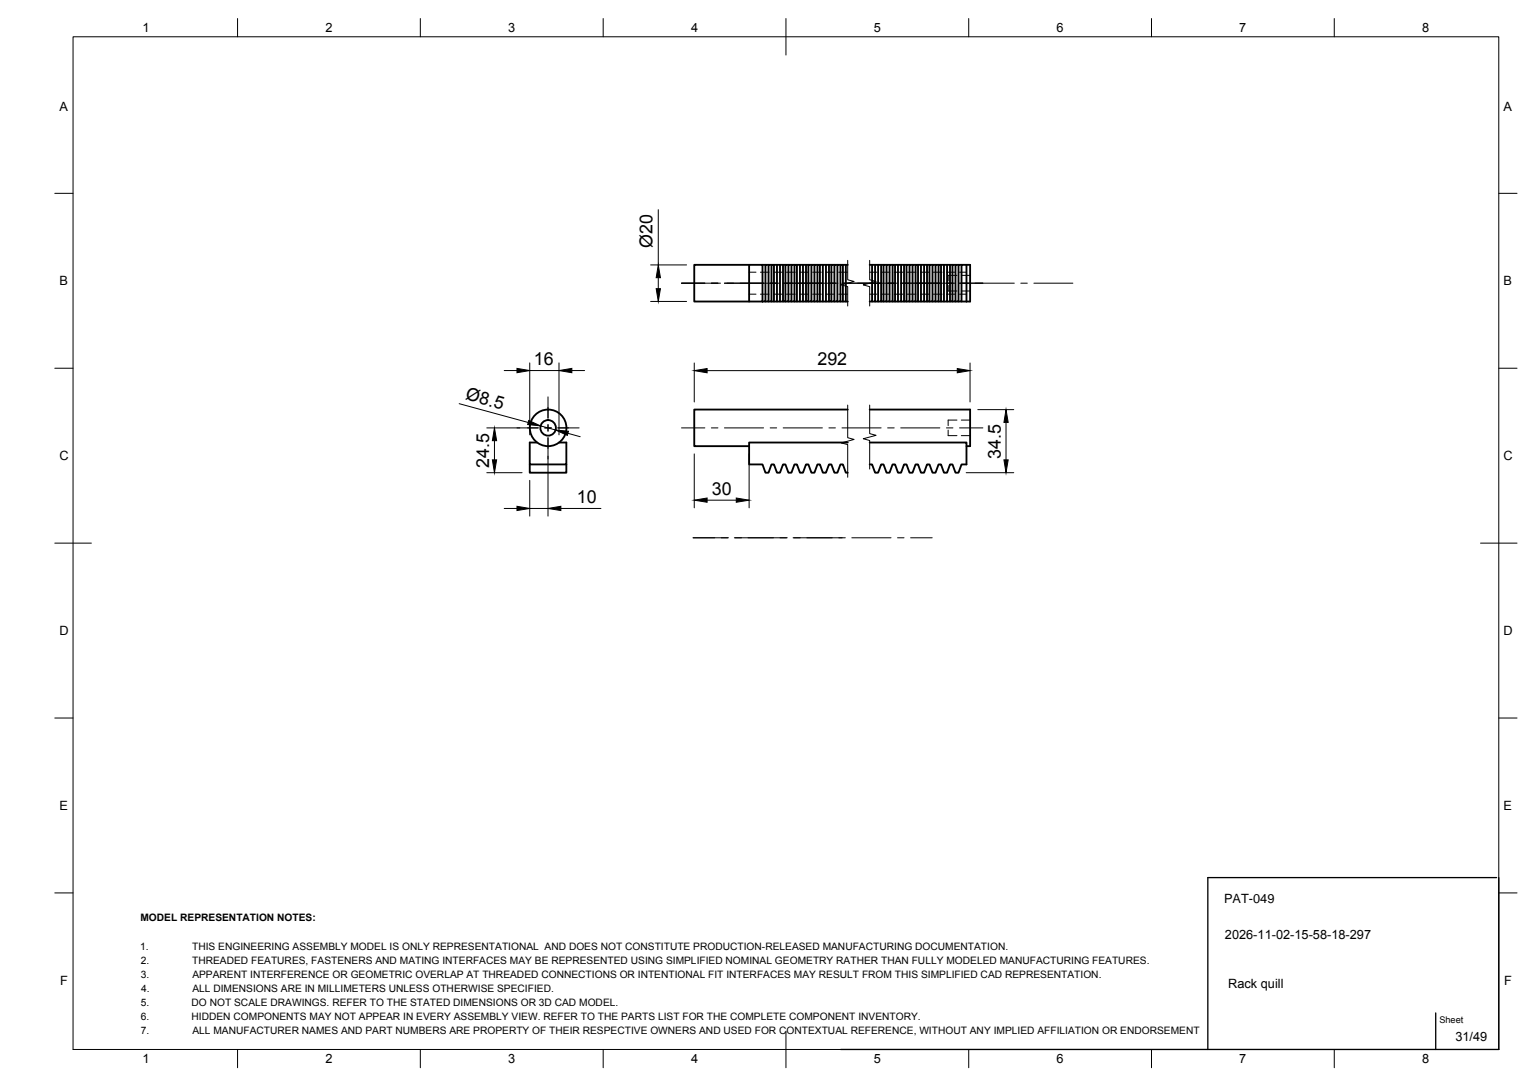
ISO-10303-21;
HEADER;
/* Generated by software containing ST-Developer
 * from STEP Tools, Inc. (www.steptools.com) 
 */

FILE_DESCRIPTION(
/* description */ ('Hand drill press frame (manual)'),
/* implementation_level */ '2;1');

FILE_NAME(
/* name */ 'Rack quill.step',
/* time_stamp */ '2026-10-28T03:25:28-07:00',
/* author */ (''),
/* organization */ (''),
/* preprocessor_version */ 'ST-DEVELOPER v20.2',
/* originating_system */ 'Autodesk Translation Framework v15.17.0.0',
/* authorisation */ '');

FILE_SCHEMA (('AUTOMOTIVE_DESIGN { 1 0 10303 214 3 1 1 }'));
ENDSEC;

DATA;
#10=MECHANICAL_DESIGN_GEOMETRIC_PRESENTATION_REPRESENTATION('',(#649),#33299);
#552=SHAPE_REPRESENTATION_RELATIONSHIP('SRR','None',#33513,#597);
#597=ADVANCED_BREP_SHAPE_REPRESENTATION('',(#700),#33275);
#649=STYLED_ITEM('',(#33800),#700);
#700=MANIFOLD_SOLID_BREP('Body1',#12668);
#846=FACE_BOUND('',#2607,.T.);
#1044=PLANE('',#13760);
#1045=PLANE('',#13761);
#1046=PLANE('',#13762);
#1047=PLANE('',#13763);
#1048=PLANE('',#13766);
#1049=PLANE('',#13769);
#1050=PLANE('',#13770);
#1051=PLANE('',#13771);
#1052=PLANE('',#13772);
#1053=PLANE('',#13773);
#1054=PLANE('',#13774);
#1055=PLANE('',#13775);
#1056=PLANE('',#13776);
#1057=PLANE('',#13777);
#1058=PLANE('',#13778);
#1059=PLANE('',#13779);
#1060=PLANE('',#13780);
#1061=PLANE('',#13781);
#1062=PLANE('',#13782);
#1063=PLANE('',#13783);
#1064=PLANE('',#13784);
#1065=PLANE('',#13785);
#1066=PLANE('',#13786);
#1067=PLANE('',#13787);
#1068=PLANE('',#13788);
#1069=PLANE('',#13789);
#1070=PLANE('',#13790);
#1071=PLANE('',#13791);
#1072=PLANE('',#13792);
#1073=PLANE('',#13793);
#1074=PLANE('',#13794);
#1075=PLANE('',#13795);
#1076=PLANE('',#13796);
#1077=PLANE('',#13797);
#1078=PLANE('',#13798);
#1079=PLANE('',#13799);
#1080=PLANE('',#13800);
#1081=PLANE('',#13801);
#1082=PLANE('',#13802);
#1083=PLANE('',#13803);
#1084=PLANE('',#13804);
#1085=PLANE('',#13805);
#1086=PLANE('',#13806);
#1087=PLANE('',#13807);
#1088=PLANE('',#13808);
#1089=PLANE('',#13809);
#1090=PLANE('',#13810);
#1091=PLANE('',#13811);
#1092=PLANE('',#13812);
#1093=PLANE('',#13813);
#1094=PLANE('',#13814);
#1095=PLANE('',#13815);
#1096=PLANE('',#13816);
#1097=PLANE('',#13817);
#1098=PLANE('',#13818);
#1099=PLANE('',#13819);
#1100=PLANE('',#13820);
#1101=PLANE('',#13821);
#1102=PLANE('',#13822);
#1103=PLANE('',#13823);
#1104=PLANE('',#13824);
#1105=PLANE('',#13825);
#1106=PLANE('',#13826);
#1107=PLANE('',#13827);
#1108=PLANE('',#13828);
#1109=PLANE('',#13829);
#1110=PLANE('',#13830);
#1111=PLANE('',#13831);
#1112=PLANE('',#13832);
#1113=PLANE('',#13833);
#1114=PLANE('',#13834);
#1115=PLANE('',#13835);
#1116=PLANE('',#13836);
#1117=PLANE('',#13837);
#1118=PLANE('',#13838);
#1119=PLANE('',#13839);
#1120=PLANE('',#13840);
#1121=PLANE('',#13841);
#1122=PLANE('',#13842);
#1123=PLANE('',#13843);
#1124=PLANE('',#13844);
#1125=PLANE('',#13845);
#1126=PLANE('',#13846);
#1127=PLANE('',#13847);
#1128=PLANE('',#13848);
#1129=PLANE('',#13849);
#1130=PLANE('',#13850);
#1131=PLANE('',#13851);
#1132=PLANE('',#13852);
#1133=PLANE('',#13853);
#1134=PLANE('',#13854);
#1135=PLANE('',#13855);
#1136=PLANE('',#13856);
#1137=PLANE('',#13857);
#1138=PLANE('',#13858);
#1139=PLANE('',#13859);
#1140=PLANE('',#13860);
#1141=PLANE('',#13861);
#1142=PLANE('',#13862);
#1143=PLANE('',#13863);
#1144=PLANE('',#13864);
#1145=PLANE('',#13865);
#1146=PLANE('',#13866);
#1147=PLANE('',#13867);
#1148=PLANE('',#13868);
#1149=PLANE('',#13869);
#1150=PLANE('',#13870);
#1151=PLANE('',#13871);
#1152=PLANE('',#13872);
#1153=PLANE('',#13873);
#1154=PLANE('',#13874);
#1155=PLANE('',#13875);
#1156=PLANE('',#13876);
#1157=PLANE('',#13877);
#1158=PLANE('',#13878);
#1159=PLANE('',#13879);
#1160=PLANE('',#13880);
#1161=PLANE('',#13881);
#1162=PLANE('',#13882);
#1163=PLANE('',#13883);
#1164=PLANE('',#13884);
#1165=PLANE('',#13885);
#1166=PLANE('',#13886);
#1167=PLANE('',#13887);
#1168=PLANE('',#13888);
#1169=PLANE('',#13889);
#1170=PLANE('',#13890);
#1171=PLANE('',#13891);
#1172=PLANE('',#13892);
#1173=PLANE('',#13893);
#1174=PLANE('',#13894);
#1175=PLANE('',#13895);
#1176=PLANE('',#13896);
#1177=PLANE('',#13897);
#1178=PLANE('',#13898);
#1179=PLANE('',#13899);
#1180=PLANE('',#13900);
#1181=PLANE('',#13901);
#1182=PLANE('',#13902);
#1183=PLANE('',#13903);
#1184=PLANE('',#13904);
#1185=PLANE('',#13905);
#1186=PLANE('',#13906);
#1187=PLANE('',#13907);
#1188=PLANE('',#13908);
#1189=PLANE('',#13909);
#1190=PLANE('',#13910);
#1191=PLANE('',#13911);
#1192=PLANE('',#13912);
#1193=PLANE('',#13913);
#1194=PLANE('',#13914);
#1195=PLANE('',#13915);
#1196=PLANE('',#13916);
#1197=PLANE('',#13917);
#1198=PLANE('',#13918);
#1199=PLANE('',#13919);
#1200=PLANE('',#13920);
#1201=PLANE('',#13921);
#1202=PLANE('',#13922);
#1203=PLANE('',#13923);
#1204=PLANE('',#13924);
#1205=PLANE('',#13925);
#1206=PLANE('',#13926);
#1207=PLANE('',#13927);
#1208=PLANE('',#13928);
#1209=PLANE('',#13929);
#1210=PLANE('',#13930);
#1211=PLANE('',#13931);
#1212=PLANE('',#13935);
#1213=PLANE('',#13936);
#1620=FACE_OUTER_BOUND('',#2435,.T.);
#1621=FACE_OUTER_BOUND('',#2436,.T.);
#1622=FACE_OUTER_BOUND('',#2437,.T.);
#1623=FACE_OUTER_BOUND('',#2438,.T.);
#1624=FACE_OUTER_BOUND('',#2439,.T.);
#1625=FACE_OUTER_BOUND('',#2440,.T.);
#1626=FACE_OUTER_BOUND('',#2441,.T.);
#1627=FACE_OUTER_BOUND('',#2442,.T.);
#1628=FACE_OUTER_BOUND('',#2443,.T.);
#1629=FACE_OUTER_BOUND('',#2444,.T.);
#1630=FACE_OUTER_BOUND('',#2445,.T.);
#1631=FACE_OUTER_BOUND('',#2446,.T.);
#1632=FACE_OUTER_BOUND('',#2447,.T.);
#1633=FACE_OUTER_BOUND('',#2448,.T.);
#1634=FACE_OUTER_BOUND('',#2449,.T.);
#1635=FACE_OUTER_BOUND('',#2450,.T.);
#1636=FACE_OUTER_BOUND('',#2451,.T.);
#1637=FACE_OUTER_BOUND('',#2452,.T.);
#1638=FACE_OUTER_BOUND('',#2453,.T.);
#1639=FACE_OUTER_BOUND('',#2454,.T.);
#1640=FACE_OUTER_BOUND('',#2455,.T.);
#1641=FACE_OUTER_BOUND('',#2456,.T.);
#1642=FACE_OUTER_BOUND('',#2457,.T.);
#1643=FACE_OUTER_BOUND('',#2458,.T.);
#1644=FACE_OUTER_BOUND('',#2459,.T.);
#1645=FACE_OUTER_BOUND('',#2460,.T.);
#1646=FACE_OUTER_BOUND('',#2461,.T.);
#1647=FACE_OUTER_BOUND('',#2462,.T.);
#1648=FACE_OUTER_BOUND('',#2463,.T.);
#1649=FACE_OUTER_BOUND('',#2464,.T.);
#1650=FACE_OUTER_BOUND('',#2465,.T.);
#1651=FACE_OUTER_BOUND('',#2466,.T.);
#1652=FACE_OUTER_BOUND('',#2467,.T.);
#1653=FACE_OUTER_BOUND('',#2468,.T.);
#1654=FACE_OUTER_BOUND('',#2469,.T.);
#1655=FACE_OUTER_BOUND('',#2470,.T.);
#1656=FACE_OUTER_BOUND('',#2471,.T.);
#1657=FACE_OUTER_BOUND('',#2472,.T.);
#1658=FACE_OUTER_BOUND('',#2473,.T.);
#1659=FACE_OUTER_BOUND('',#2474,.T.);
#1660=FACE_OUTER_BOUND('',#2475,.T.);
#1661=FACE_OUTER_BOUND('',#2476,.T.);
#1662=FACE_OUTER_BOUND('',#2477,.T.);
#1663=FACE_OUTER_BOUND('',#2478,.T.);
#1664=FACE_OUTER_BOUND('',#2479,.T.);
#1665=FACE_OUTER_BOUND('',#2480,.T.);
#1666=FACE_OUTER_BOUND('',#2481,.T.);
#1667=FACE_OUTER_BOUND('',#2482,.T.);
#1668=FACE_OUTER_BOUND('',#2483,.T.);
#1669=FACE_OUTER_BOUND('',#2484,.T.);
#1670=FACE_OUTER_BOUND('',#2485,.T.);
#1671=FACE_OUTER_BOUND('',#2486,.T.);
#1672=FACE_OUTER_BOUND('',#2487,.T.);
#1673=FACE_OUTER_BOUND('',#2488,.T.);
#1674=FACE_OUTER_BOUND('',#2489,.T.);
#1675=FACE_OUTER_BOUND('',#2490,.T.);
#1676=FACE_OUTER_BOUND('',#2491,.T.);
#1677=FACE_OUTER_BOUND('',#2492,.T.);
#1678=FACE_OUTER_BOUND('',#2493,.T.);
#1679=FACE_OUTER_BOUND('',#2494,.T.);
#1680=FACE_OUTER_BOUND('',#2495,.T.);
#1681=FACE_OUTER_BOUND('',#2496,.T.);
#1682=FACE_OUTER_BOUND('',#2497,.T.);
#1683=FACE_OUTER_BOUND('',#2498,.T.);
#1684=FACE_OUTER_BOUND('',#2499,.T.);
#1685=FACE_OUTER_BOUND('',#2500,.T.);
#1686=FACE_OUTER_BOUND('',#2501,.T.);
#1687=FACE_OUTER_BOUND('',#2502,.T.);
#1688=FACE_OUTER_BOUND('',#2503,.T.);
#1689=FACE_OUTER_BOUND('',#2504,.T.);
#1690=FACE_OUTER_BOUND('',#2505,.T.);
#1691=FACE_OUTER_BOUND('',#2506,.T.);
#1692=FACE_OUTER_BOUND('',#2507,.T.);
#1693=FACE_OUTER_BOUND('',#2508,.T.);
#1694=FACE_OUTER_BOUND('',#2509,.T.);
#1695=FACE_OUTER_BOUND('',#2510,.T.);
#1696=FACE_OUTER_BOUND('',#2511,.T.);
#1697=FACE_OUTER_BOUND('',#2512,.T.);
#1698=FACE_OUTER_BOUND('',#2513,.T.);
#1699=FACE_OUTER_BOUND('',#2514,.T.);
#1700=FACE_OUTER_BOUND('',#2515,.T.);
#1701=FACE_OUTER_BOUND('',#2516,.T.);
#1702=FACE_OUTER_BOUND('',#2517,.T.);
#1703=FACE_OUTER_BOUND('',#2518,.T.);
#1704=FACE_OUTER_BOUND('',#2519,.T.);
#1705=FACE_OUTER_BOUND('',#2520,.T.);
#1706=FACE_OUTER_BOUND('',#2521,.T.);
#1707=FACE_OUTER_BOUND('',#2522,.T.);
#1708=FACE_OUTER_BOUND('',#2523,.T.);
#1709=FACE_OUTER_BOUND('',#2524,.T.);
#1710=FACE_OUTER_BOUND('',#2525,.T.);
#1711=FACE_OUTER_BOUND('',#2526,.T.);
#1712=FACE_OUTER_BOUND('',#2527,.T.);
#1713=FACE_OUTER_BOUND('',#2528,.T.);
#1714=FACE_OUTER_BOUND('',#2529,.T.);
#1715=FACE_OUTER_BOUND('',#2530,.T.);
#1716=FACE_OUTER_BOUND('',#2531,.T.);
#1717=FACE_OUTER_BOUND('',#2532,.T.);
#1718=FACE_OUTER_BOUND('',#2533,.T.);
#1719=FACE_OUTER_BOUND('',#2534,.T.);
#1720=FACE_OUTER_BOUND('',#2535,.T.);
#1721=FACE_OUTER_BOUND('',#2536,.T.);
#1722=FACE_OUTER_BOUND('',#2537,.T.);
#1723=FACE_OUTER_BOUND('',#2538,.T.);
#1724=FACE_OUTER_BOUND('',#2539,.T.);
#1725=FACE_OUTER_BOUND('',#2540,.T.);
#1726=FACE_OUTER_BOUND('',#2541,.T.);
#1727=FACE_OUTER_BOUND('',#2542,.T.);
#1728=FACE_OUTER_BOUND('',#2543,.T.);
#1729=FACE_OUTER_BOUND('',#2544,.T.);
#1730=FACE_OUTER_BOUND('',#2545,.T.);
#1731=FACE_OUTER_BOUND('',#2546,.T.);
#1732=FACE_OUTER_BOUND('',#2547,.T.);
#1733=FACE_OUTER_BOUND('',#2548,.T.);
#1734=FACE_OUTER_BOUND('',#2549,.T.);
#1735=FACE_OUTER_BOUND('',#2550,.T.);
#1736=FACE_OUTER_BOUND('',#2551,.T.);
#1737=FACE_OUTER_BOUND('',#2552,.T.);
#1738=FACE_OUTER_BOUND('',#2553,.T.);
#1739=FACE_OUTER_BOUND('',#2554,.T.);
#1740=FACE_OUTER_BOUND('',#2555,.T.);
#1741=FACE_OUTER_BOUND('',#2556,.T.);
#1742=FACE_OUTER_BOUND('',#2557,.T.);
#1743=FACE_OUTER_BOUND('',#2558,.T.);
#1744=FACE_OUTER_BOUND('',#2559,.T.);
#1745=FACE_OUTER_BOUND('',#2560,.T.);
#1746=FACE_OUTER_BOUND('',#2561,.T.);
#1747=FACE_OUTER_BOUND('',#2562,.T.);
#1748=FACE_OUTER_BOUND('',#2563,.T.);
#1749=FACE_OUTER_BOUND('',#2564,.T.);
#1750=FACE_OUTER_BOUND('',#2565,.T.);
#1751=FACE_OUTER_BOUND('',#2566,.T.);
#1752=FACE_OUTER_BOUND('',#2567,.T.);
#1753=FACE_OUTER_BOUND('',#2568,.T.);
#1754=FACE_OUTER_BOUND('',#2569,.T.);
#1755=FACE_OUTER_BOUND('',#2570,.T.);
#1756=FACE_OUTER_BOUND('',#2571,.T.);
#1757=FACE_OUTER_BOUND('',#2572,.T.);
#1758=FACE_OUTER_BOUND('',#2573,.T.);
#1759=FACE_OUTER_BOUND('',#2574,.T.);
#1760=FACE_OUTER_BOUND('',#2575,.T.);
#1761=FACE_OUTER_BOUND('',#2576,.T.);
#1762=FACE_OUTER_BOUND('',#2577,.T.);
#1763=FACE_OUTER_BOUND('',#2578,.T.);
#1764=FACE_OUTER_BOUND('',#2579,.T.);
#1765=FACE_OUTER_BOUND('',#2580,.T.);
#1766=FACE_OUTER_BOUND('',#2581,.T.);
#1767=FACE_OUTER_BOUND('',#2582,.T.);
#1768=FACE_OUTER_BOUND('',#2583,.T.);
#1769=FACE_OUTER_BOUND('',#2584,.T.);
#1770=FACE_OUTER_BOUND('',#2585,.T.);
#1771=FACE_OUTER_BOUND('',#2586,.T.);
#1772=FACE_OUTER_BOUND('',#2587,.T.);
#1773=FACE_OUTER_BOUND('',#2588,.T.);
#1774=FACE_OUTER_BOUND('',#2589,.T.);
#1775=FACE_OUTER_BOUND('',#2590,.T.);
#1776=FACE_OUTER_BOUND('',#2591,.T.);
#1777=FACE_OUTER_BOUND('',#2592,.T.);
#1778=FACE_OUTER_BOUND('',#2593,.T.);
#1779=FACE_OUTER_BOUND('',#2594,.T.);
#1780=FACE_OUTER_BOUND('',#2595,.T.);
#1781=FACE_OUTER_BOUND('',#2596,.T.);
#1782=FACE_OUTER_BOUND('',#2597,.T.);
#1783=FACE_OUTER_BOUND('',#2598,.T.);
#1784=FACE_OUTER_BOUND('',#2599,.T.);
#1785=FACE_OUTER_BOUND('',#2600,.T.);
#1786=FACE_OUTER_BOUND('',#2601,.T.);
#1787=FACE_OUTER_BOUND('',#2602,.T.);
#1788=FACE_OUTER_BOUND('',#2603,.T.);
#1789=FACE_OUTER_BOUND('',#2604,.T.);
#1790=FACE_OUTER_BOUND('',#2605,.T.);
#1791=FACE_OUTER_BOUND('',#2606,.T.);
#2435=EDGE_LOOP('',(#9705,#9706,#9707,#9708));
#2436=EDGE_LOOP('',(#9709));
#2437=EDGE_LOOP('',(#9710,#9711,#9712,#9713));
#2438=EDGE_LOOP('',(#9714,#9715,#9716,#9717));
#2439=EDGE_LOOP('',(#9718,#9719,#9720,#9721,#9722,#9723,#9724));
#2440=EDGE_LOOP('',(#9725,#9726,#9727,#9728,#9729,#9730,#9731));
#2441=EDGE_LOOP('',(#9732,#9733,#9734,#9735));
#2442=EDGE_LOOP('',(#9736,#9737,#9738,#9739));
#2443=EDGE_LOOP('',(#9740,#9741,#9742,#9743));
#2444=EDGE_LOOP('',(#9744,#9745,#9746,#9747));
#2445=EDGE_LOOP('',(#9748,#9749,#9750,#9751));
#2446=EDGE_LOOP('',(#9752,#9753,#9754,#9755));
#2447=EDGE_LOOP('',(#9756,#9757,#9758,#9759));
#2448=EDGE_LOOP('',(#9760,#9761,#9762,#9763));
#2449=EDGE_LOOP('',(#9764,#9765,#9766,#9767));
#2450=EDGE_LOOP('',(#9768,#9769,#9770,#9771));
#2451=EDGE_LOOP('',(#9772,#9773,#9774,#9775));
#2452=EDGE_LOOP('',(#9776,#9777,#9778,#9779));
#2453=EDGE_LOOP('',(#9780,#9781,#9782,#9783));
#2454=EDGE_LOOP('',(#9784,#9785,#9786,#9787));
#2455=EDGE_LOOP('',(#9788,#9789,#9790,#9791));
#2456=EDGE_LOOP('',(#9792,#9793,#9794,#9795));
#2457=EDGE_LOOP('',(#9796,#9797,#9798,#9799));
#2458=EDGE_LOOP('',(#9800,#9801,#9802,#9803));
#2459=EDGE_LOOP('',(#9804,#9805,#9806,#9807));
#2460=EDGE_LOOP('',(#9808,#9809,#9810,#9811));
#2461=EDGE_LOOP('',(#9812,#9813,#9814,#9815));
#2462=EDGE_LOOP('',(#9816,#9817,#9818,#9819));
#2463=EDGE_LOOP('',(#9820,#9821,#9822,#9823));
#2464=EDGE_LOOP('',(#9824,#9825,#9826,#9827));
#2465=EDGE_LOOP('',(#9828,#9829,#9830,#9831));
#2466=EDGE_LOOP('',(#9832,#9833,#9834,#9835));
#2467=EDGE_LOOP('',(#9836,#9837,#9838,#9839));
#2468=EDGE_LOOP('',(#9840,#9841,#9842,#9843));
#2469=EDGE_LOOP('',(#9844,#9845,#9846,#9847));
#2470=EDGE_LOOP('',(#9848,#9849,#9850,#9851));
#2471=EDGE_LOOP('',(#9852,#9853,#9854,#9855));
#2472=EDGE_LOOP('',(#9856,#9857,#9858,#9859));
#2473=EDGE_LOOP('',(#9860,#9861,#9862,#9863));
#2474=EDGE_LOOP('',(#9864,#9865,#9866,#9867));
#2475=EDGE_LOOP('',(#9868,#9869,#9870,#9871));
#2476=EDGE_LOOP('',(#9872,#9873,#9874,#9875));
#2477=EDGE_LOOP('',(#9876,#9877,#9878,#9879));
#2478=EDGE_LOOP('',(#9880,#9881,#9882,#9883));
#2479=EDGE_LOOP('',(#9884,#9885,#9886,#9887));
#2480=EDGE_LOOP('',(#9888,#9889,#9890,#9891));
#2481=EDGE_LOOP('',(#9892,#9893,#9894,#9895));
#2482=EDGE_LOOP('',(#9896,#9897,#9898,#9899));
#2483=EDGE_LOOP('',(#9900,#9901,#9902,#9903));
#2484=EDGE_LOOP('',(#9904,#9905,#9906,#9907));
#2485=EDGE_LOOP('',(#9908,#9909,#9910,#9911));
#2486=EDGE_LOOP('',(#9912,#9913,#9914,#9915));
#2487=EDGE_LOOP('',(#9916,#9917,#9918,#9919));
#2488=EDGE_LOOP('',(#9920,#9921,#9922,#9923));
#2489=EDGE_LOOP('',(#9924,#9925,#9926,#9927));
#2490=EDGE_LOOP('',(#9928,#9929,#9930,#9931));
#2491=EDGE_LOOP('',(#9932,#9933,#9934,#9935));
#2492=EDGE_LOOP('',(#9936,#9937,#9938,#9939));
#2493=EDGE_LOOP('',(#9940,#9941,#9942,#9943));
#2494=EDGE_LOOP('',(#9944,#9945,#9946,#9947));
#2495=EDGE_LOOP('',(#9948,#9949,#9950,#9951));
#2496=EDGE_LOOP('',(#9952,#9953,#9954,#9955));
#2497=EDGE_LOOP('',(#9956,#9957,#9958,#9959));
#2498=EDGE_LOOP('',(#9960,#9961,#9962,#9963));
#2499=EDGE_LOOP('',(#9964,#9965,#9966,#9967));
#2500=EDGE_LOOP('',(#9968,#9969,#9970,#9971));
#2501=EDGE_LOOP('',(#9972,#9973,#9974,#9975));
#2502=EDGE_LOOP('',(#9976,#9977,#9978,#9979));
#2503=EDGE_LOOP('',(#9980,#9981,#9982,#9983));
#2504=EDGE_LOOP('',(#9984,#9985,#9986,#9987));
#2505=EDGE_LOOP('',(#9988,#9989,#9990,#9991));
#2506=EDGE_LOOP('',(#9992,#9993,#9994,#9995));
#2507=EDGE_LOOP('',(#9996,#9997,#9998,#9999));
#2508=EDGE_LOOP('',(#10000,#10001,#10002,#10003));
#2509=EDGE_LOOP('',(#10004,#10005,#10006,#10007));
#2510=EDGE_LOOP('',(#10008,#10009,#10010,#10011));
#2511=EDGE_LOOP('',(#10012,#10013,#10014,#10015));
#2512=EDGE_LOOP('',(#10016,#10017,#10018,#10019));
#2513=EDGE_LOOP('',(#10020,#10021,#10022,#10023));
#2514=EDGE_LOOP('',(#10024,#10025,#10026,#10027));
#2515=EDGE_LOOP('',(#10028,#10029,#10030,#10031));
#2516=EDGE_LOOP('',(#10032,#10033,#10034,#10035));
#2517=EDGE_LOOP('',(#10036,#10037,#10038,#10039));
#2518=EDGE_LOOP('',(#10040,#10041,#10042,#10043));
#2519=EDGE_LOOP('',(#10044,#10045,#10046,#10047));
#2520=EDGE_LOOP('',(#10048,#10049,#10050,#10051));
#2521=EDGE_LOOP('',(#10052,#10053,#10054,#10055));
#2522=EDGE_LOOP('',(#10056,#10057,#10058,#10059));
#2523=EDGE_LOOP('',(#10060,#10061,#10062,#10063));
#2524=EDGE_LOOP('',(#10064,#10065,#10066,#10067));
#2525=EDGE_LOOP('',(#10068,#10069,#10070,#10071));
#2526=EDGE_LOOP('',(#10072,#10073,#10074,#10075));
#2527=EDGE_LOOP('',(#10076,#10077,#10078,#10079));
#2528=EDGE_LOOP('',(#10080,#10081,#10082,#10083));
#2529=EDGE_LOOP('',(#10084,#10085,#10086,#10087));
#2530=EDGE_LOOP('',(#10088,#10089,#10090,#10091));
#2531=EDGE_LOOP('',(#10092,#10093,#10094,#10095));
#2532=EDGE_LOOP('',(#10096,#10097,#10098,#10099));
#2533=EDGE_LOOP('',(#10100,#10101,#10102,#10103));
#2534=EDGE_LOOP('',(#10104,#10105,#10106,#10107));
#2535=EDGE_LOOP('',(#10108,#10109,#10110,#10111));
#2536=EDGE_LOOP('',(#10112,#10113,#10114,#10115));
#2537=EDGE_LOOP('',(#10116,#10117,#10118,#10119));
#2538=EDGE_LOOP('',(#10120,#10121,#10122,#10123));
#2539=EDGE_LOOP('',(#10124,#10125,#10126,#10127));
#2540=EDGE_LOOP('',(#10128,#10129,#10130,#10131));
#2541=EDGE_LOOP('',(#10132,#10133,#10134,#10135));
#2542=EDGE_LOOP('',(#10136,#10137,#10138,#10139));
#2543=EDGE_LOOP('',(#10140,#10141,#10142,#10143));
#2544=EDGE_LOOP('',(#10144,#10145,#10146,#10147));
#2545=EDGE_LOOP('',(#10148,#10149,#10150,#10151));
#2546=EDGE_LOOP('',(#10152,#10153,#10154,#10155));
#2547=EDGE_LOOP('',(#10156,#10157,#10158,#10159));
#2548=EDGE_LOOP('',(#10160,#10161,#10162,#10163));
#2549=EDGE_LOOP('',(#10164,#10165,#10166,#10167));
#2550=EDGE_LOOP('',(#10168,#10169,#10170,#10171));
#2551=EDGE_LOOP('',(#10172,#10173,#10174,#10175));
#2552=EDGE_LOOP('',(#10176,#10177,#10178,#10179));
#2553=EDGE_LOOP('',(#10180,#10181,#10182,#10183));
#2554=EDGE_LOOP('',(#10184,#10185,#10186,#10187));
#2555=EDGE_LOOP('',(#10188,#10189,#10190,#10191));
#2556=EDGE_LOOP('',(#10192,#10193,#10194,#10195));
#2557=EDGE_LOOP('',(#10196,#10197,#10198,#10199));
#2558=EDGE_LOOP('',(#10200,#10201,#10202,#10203));
#2559=EDGE_LOOP('',(#10204,#10205,#10206,#10207));
#2560=EDGE_LOOP('',(#10208,#10209,#10210,#10211));
#2561=EDGE_LOOP('',(#10212,#10213,#10214,#10215));
#2562=EDGE_LOOP('',(#10216,#10217,#10218,#10219));
#2563=EDGE_LOOP('',(#10220,#10221,#10222,#10223));
#2564=EDGE_LOOP('',(#10224,#10225,#10226,#10227));
#2565=EDGE_LOOP('',(#10228,#10229,#10230,#10231));
#2566=EDGE_LOOP('',(#10232,#10233,#10234,#10235));
#2567=EDGE_LOOP('',(#10236,#10237,#10238,#10239));
#2568=EDGE_LOOP('',(#10240,#10241,#10242,#10243));
#2569=EDGE_LOOP('',(#10244,#10245,#10246,#10247));
#2570=EDGE_LOOP('',(#10248,#10249,#10250,#10251));
#2571=EDGE_LOOP('',(#10252,#10253,#10254,#10255));
#2572=EDGE_LOOP('',(#10256,#10257,#10258,#10259));
#2573=EDGE_LOOP('',(#10260,#10261,#10262,#10263));
#2574=EDGE_LOOP('',(#10264,#10265,#10266,#10267));
#2575=EDGE_LOOP('',(#10268,#10269,#10270,#10271));
#2576=EDGE_LOOP('',(#10272,#10273,#10274,#10275));
#2577=EDGE_LOOP('',(#10276,#10277,#10278,#10279));
#2578=EDGE_LOOP('',(#10280,#10281,#10282,#10283));
#2579=EDGE_LOOP('',(#10284,#10285,#10286,#10287));
#2580=EDGE_LOOP('',(#10288,#10289,#10290,#10291));
#2581=EDGE_LOOP('',(#10292,#10293,#10294,#10295));
#2582=EDGE_LOOP('',(#10296,#10297,#10298,#10299));
#2583=EDGE_LOOP('',(#10300,#10301,#10302,#10303));
#2584=EDGE_LOOP('',(#10304,#10305,#10306,#10307));
#2585=EDGE_LOOP('',(#10308,#10309,#10310,#10311));
#2586=EDGE_LOOP('',(#10312,#10313,#10314,#10315));
#2587=EDGE_LOOP('',(#10316,#10317,#10318,#10319));
#2588=EDGE_LOOP('',(#10320,#10321,#10322,#10323));
#2589=EDGE_LOOP('',(#10324,#10325,#10326,#10327));
#2590=EDGE_LOOP('',(#10328,#10329,#10330,#10331));
#2591=EDGE_LOOP('',(#10332,#10333,#10334,#10335));
#2592=EDGE_LOOP('',(#10336,#10337,#10338,#10339));
#2593=EDGE_LOOP('',(#10340,#10341,#10342,#10343));
#2594=EDGE_LOOP('',(#10344,#10345,#10346,#10347));
#2595=EDGE_LOOP('',(#10348,#10349,#10350,#10351));
#2596=EDGE_LOOP('',(#10352,#10353,#10354,#10355));
#2597=EDGE_LOOP('',(#10356,#10357,#10358,#10359));
#2598=EDGE_LOOP('',(#10360,#10361,#10362,#10363));
#2599=EDGE_LOOP('',(#10364,#10365,#10366,#10367));
#2600=EDGE_LOOP('',(#10368,#10369,#10370,#10371));
#2601=EDGE_LOOP('',(#10372,#10373,#10374,#10375));
#2602=EDGE_LOOP('',(#10376,#10377,#10378,#10379,#10380,#10381,#10382,#10383,
#10384,#10385,#10386,#10387,#10388,#10389,#10390,#10391,#10392,#10393,#10394,
#10395,#10396,#10397,#10398,#10399,#10400,#10401,#10402,#10403,#10404,#10405,
#10406,#10407,#10408,#10409,#10410,#10411,#10412,#10413,#10414,#10415,#10416,
#10417,#10418,#10419,#10420,#10421,#10422,#10423,#10424,#10425,#10426,#10427,
#10428,#10429,#10430,#10431,#10432,#10433,#10434,#10435,#10436,#10437,#10438,
#10439,#10440,#10441,#10442,#10443,#10444,#10445,#10446,#10447,#10448,#10449,
#10450,#10451,#10452,#10453,#10454,#10455,#10456,#10457,#10458,#10459,#10460,
#10461,#10462,#10463,#10464,#10465,#10466,#10467,#10468,#10469,#10470,#10471,
#10472,#10473,#10474,#10475,#10476,#10477,#10478,#10479,#10480,#10481,#10482,
#10483,#10484,#10485,#10486,#10487,#10488,#10489,#10490,#10491,#10492,#10493,
#10494,#10495,#10496,#10497,#10498,#10499,#10500,#10501,#10502,#10503,#10504,
#10505,#10506,#10507,#10508,#10509,#10510,#10511,#10512,#10513,#10514,#10515,
#10516,#10517,#10518,#10519,#10520,#10521,#10522,#10523,#10524,#10525,#10526,
#10527,#10528,#10529,#10530,#10531,#10532,#10533,#10534,#10535,#10536,#10537,
#10538,#10539));
#2603=EDGE_LOOP('',(#10540,#10541,#10542,#10543,#10544,#10545,#10546,#10547,
#10548,#10549,#10550,#10551,#10552,#10553,#10554,#10555,#10556,#10557,#10558,
#10559,#10560,#10561,#10562,#10563,#10564,#10565,#10566,#10567,#10568,#10569,
#10570,#10571,#10572,#10573,#10574,#10575,#10576,#10577,#10578,#10579,#10580,
#10581,#10582,#10583,#10584,#10585,#10586,#10587,#10588,#10589,#10590,#10591,
#10592,#10593,#10594,#10595,#10596,#10597,#10598,#10599,#10600,#10601,#10602,
#10603,#10604,#10605,#10606,#10607,#10608,#10609,#10610,#10611,#10612,#10613,
#10614,#10615,#10616,#10617,#10618,#10619,#10620,#10621,#10622,#10623,#10624,
#10625,#10626,#10627,#10628,#10629,#10630,#10631,#10632,#10633,#10634,#10635,
#10636,#10637,#10638,#10639,#10640,#10641,#10642,#10643,#10644,#10645,#10646,
#10647,#10648,#10649,#10650,#10651,#10652,#10653,#10654,#10655,#10656,#10657,
#10658,#10659,#10660,#10661,#10662,#10663,#10664,#10665,#10666,#10667,#10668,
#10669,#10670,#10671,#10672,#10673,#10674,#10675,#10676,#10677,#10678,#10679,
#10680,#10681,#10682,#10683,#10684,#10685,#10686,#10687,#10688,#10689,#10690,
#10691,#10692,#10693,#10694,#10695,#10696,#10697,#10698,#10699,#10700,#10701,
#10702,#10703));
#2604=EDGE_LOOP('',(#10704,#10705,#10706,#10707,#10708,#10709,#10710,#10711,
#10712,#10713,#10714,#10715));
#2605=EDGE_LOOP('',(#10716));
#2606=EDGE_LOOP('',(#10717));
#2607=EDGE_LOOP('',(#10718));
#3242=LINE('',#19762,#4407);
#3243=LINE('',#19768,#4408);
#3244=LINE('',#19770,#4409);
#3245=LINE('',#19772,#4410);
#3246=LINE('',#19773,#4411);
#3247=LINE('',#19777,#4412);
#3248=LINE('',#19779,#4413);
#3249=LINE('',#19781,#4414);
#3250=LINE('',#19782,#4415);
#3251=LINE('',#19787,#4416);
#3252=LINE('',#19789,#4417);
#3253=LINE('',#19790,#4418);
#3254=LINE('',#19796,#4419);
#3255=LINE('',#19798,#4420);
#3256=LINE('',#19799,#4421);
#3257=LINE('',#19803,#4422);
#3258=LINE('',#19805,#4423);
#3259=LINE('',#19806,#4424);
#3260=LINE('',#19809,#4425);
#3261=LINE('',#19811,#4426);
#3262=LINE('',#19812,#4427);
#3263=LINE('',#19815,#4428);
#3264=LINE('',#19817,#4429);
#3265=LINE('',#19818,#4430);
#3266=LINE('',#19821,#4431);
#3267=LINE('',#19823,#4432);
#3268=LINE('',#19824,#4433);
#3269=LINE('',#19827,#4434);
#3270=LINE('',#19829,#4435);
#3271=LINE('',#19830,#4436);
#3272=LINE('',#19833,#4437);
#3273=LINE('',#19835,#4438);
#3274=LINE('',#19836,#4439);
#3275=LINE('',#19839,#4440);
#3276=LINE('',#19841,#4441);
#3277=LINE('',#19842,#4442);
#3278=LINE('',#19845,#4443);
#3279=LINE('',#19847,#4444);
#3280=LINE('',#19848,#4445);
#3281=LINE('',#19851,#4446);
#3282=LINE('',#19853,#4447);
#3283=LINE('',#19854,#4448);
#3284=LINE('',#19857,#4449);
#3285=LINE('',#19859,#4450);
#3286=LINE('',#19860,#4451);
#3287=LINE('',#19863,#4452);
#3288=LINE('',#19865,#4453);
#3289=LINE('',#19866,#4454);
#3290=LINE('',#19869,#4455);
#3291=LINE('',#19871,#4456);
#3292=LINE('',#19872,#4457);
#3293=LINE('',#19875,#4458);
#3294=LINE('',#19877,#4459);
#3295=LINE('',#19878,#4460);
#3296=LINE('',#19881,#4461);
#3297=LINE('',#19883,#4462);
#3298=LINE('',#19884,#4463);
#3299=LINE('',#19887,#4464);
#3300=LINE('',#19889,#4465);
#3301=LINE('',#19890,#4466);
#3302=LINE('',#19893,#4467);
#3303=LINE('',#19895,#4468);
#3304=LINE('',#19896,#4469);
#3305=LINE('',#19899,#4470);
#3306=LINE('',#19901,#4471);
#3307=LINE('',#19902,#4472);
#3308=LINE('',#19905,#4473);
#3309=LINE('',#19907,#4474);
#3310=LINE('',#19908,#4475);
#3311=LINE('',#19911,#4476);
#3312=LINE('',#19913,#4477);
#3313=LINE('',#19914,#4478);
#3314=LINE('',#19917,#4479);
#3315=LINE('',#19919,#4480);
#3316=LINE('',#19920,#4481);
#3317=LINE('',#19923,#4482);
#3318=LINE('',#19925,#4483);
#3319=LINE('',#19926,#4484);
#3320=LINE('',#19929,#4485);
#3321=LINE('',#19931,#4486);
#3322=LINE('',#19932,#4487);
#3323=LINE('',#19935,#4488);
#3324=LINE('',#19937,#4489);
#3325=LINE('',#19938,#4490);
#3326=LINE('',#19941,#4491);
#3327=LINE('',#19943,#4492);
#3328=LINE('',#19944,#4493);
#3329=LINE('',#19947,#4494);
#3330=LINE('',#19949,#4495);
#3331=LINE('',#19950,#4496);
#3332=LINE('',#19953,#4497);
#3333=LINE('',#19955,#4498);
#3334=LINE('',#19956,#4499);
#3335=LINE('',#19959,#4500);
#3336=LINE('',#19961,#4501);
#3337=LINE('',#19962,#4502);
#3338=LINE('',#19965,#4503);
#3339=LINE('',#19967,#4504);
#3340=LINE('',#19968,#4505);
#3341=LINE('',#19971,#4506);
#3342=LINE('',#19973,#4507);
#3343=LINE('',#19974,#4508);
#3344=LINE('',#19977,#4509);
#3345=LINE('',#19979,#4510);
#3346=LINE('',#19980,#4511);
#3347=LINE('',#19983,#4512);
#3348=LINE('',#19985,#4513);
#3349=LINE('',#19986,#4514);
#3350=LINE('',#19989,#4515);
#3351=LINE('',#19991,#4516);
#3352=LINE('',#19992,#4517);
#3353=LINE('',#19995,#4518);
#3354=LINE('',#19997,#4519);
#3355=LINE('',#19998,#4520);
#3356=LINE('',#20001,#4521);
#3357=LINE('',#20003,#4522);
#3358=LINE('',#20004,#4523);
#3359=LINE('',#20007,#4524);
#3360=LINE('',#20009,#4525);
#3361=LINE('',#20010,#4526);
#3362=LINE('',#20013,#4527);
#3363=LINE('',#20015,#4528);
#3364=LINE('',#20016,#4529);
#3365=LINE('',#20019,#4530);
#3366=LINE('',#20021,#4531);
#3367=LINE('',#20022,#4532);
#3368=LINE('',#20025,#4533);
#3369=LINE('',#20027,#4534);
#3370=LINE('',#20028,#4535);
#3371=LINE('',#20031,#4536);
#3372=LINE('',#20033,#4537);
#3373=LINE('',#20034,#4538);
#3374=LINE('',#20037,#4539);
#3375=LINE('',#20039,#4540);
#3376=LINE('',#20040,#4541);
#3377=LINE('',#20043,#4542);
#3378=LINE('',#20045,#4543);
#3379=LINE('',#20046,#4544);
#3380=LINE('',#20049,#4545);
#3381=LINE('',#20051,#4546);
#3382=LINE('',#20052,#4547);
#3383=LINE('',#20055,#4548);
#3384=LINE('',#20057,#4549);
#3385=LINE('',#20058,#4550);
#3386=LINE('',#20061,#4551);
#3387=LINE('',#20063,#4552);
#3388=LINE('',#20064,#4553);
#3389=LINE('',#20067,#4554);
#3390=LINE('',#20069,#4555);
#3391=LINE('',#20070,#4556);
#3392=LINE('',#20073,#4557);
#3393=LINE('',#20075,#4558);
#3394=LINE('',#20076,#4559);
#3395=LINE('',#20079,#4560);
#3396=LINE('',#20081,#4561);
#3397=LINE('',#20082,#4562);
#3398=LINE('',#20085,#4563);
#3399=LINE('',#20087,#4564);
#3400=LINE('',#20088,#4565);
#3401=LINE('',#20091,#4566);
#3402=LINE('',#20093,#4567);
#3403=LINE('',#20094,#4568);
#3404=LINE('',#20097,#4569);
#3405=LINE('',#20099,#4570);
#3406=LINE('',#20100,#4571);
#3407=LINE('',#20103,#4572);
#3408=LINE('',#20105,#4573);
#3409=LINE('',#20106,#4574);
#3410=LINE('',#20109,#4575);
#3411=LINE('',#20111,#4576);
#3412=LINE('',#20112,#4577);
#3413=LINE('',#20115,#4578);
#3414=LINE('',#20117,#4579);
#3415=LINE('',#20118,#4580);
#3416=LINE('',#20121,#4581);
#3417=LINE('',#20123,#4582);
#3418=LINE('',#20124,#4583);
#3419=LINE('',#20127,#4584);
#3420=LINE('',#20129,#4585);
#3421=LINE('',#20130,#4586);
#3422=LINE('',#20133,#4587);
#3423=LINE('',#20135,#4588);
#3424=LINE('',#20136,#4589);
#3425=LINE('',#20139,#4590);
#3426=LINE('',#20141,#4591);
#3427=LINE('',#20142,#4592);
#3428=LINE('',#20145,#4593);
#3429=LINE('',#20147,#4594);
#3430=LINE('',#20148,#4595);
#3431=LINE('',#20151,#4596);
#3432=LINE('',#20153,#4597);
#3433=LINE('',#20154,#4598);
#3434=LINE('',#20157,#4599);
#3435=LINE('',#20159,#4600);
#3436=LINE('',#20160,#4601);
#3437=LINE('',#20163,#4602);
#3438=LINE('',#20165,#4603);
#3439=LINE('',#20166,#4604);
#3440=LINE('',#20169,#4605);
#3441=LINE('',#20171,#4606);
#3442=LINE('',#20172,#4607);
#3443=LINE('',#20175,#4608);
#3444=LINE('',#20177,#4609);
#3445=LINE('',#20178,#4610);
#3446=LINE('',#20181,#4611);
#3447=LINE('',#20183,#4612);
#3448=LINE('',#20184,#4613);
#3449=LINE('',#20187,#4614);
#3450=LINE('',#20189,#4615);
#3451=LINE('',#20190,#4616);
#3452=LINE('',#20193,#4617);
#3453=LINE('',#20195,#4618);
#3454=LINE('',#20196,#4619);
#3455=LINE('',#20199,#4620);
#3456=LINE('',#20201,#4621);
#3457=LINE('',#20202,#4622);
#3458=LINE('',#20205,#4623);
#3459=LINE('',#20207,#4624);
#3460=LINE('',#20208,#4625);
#3461=LINE('',#20211,#4626);
#3462=LINE('',#20213,#4627);
#3463=LINE('',#20214,#4628);
#3464=LINE('',#20217,#4629);
#3465=LINE('',#20219,#4630);
#3466=LINE('',#20220,#4631);
#3467=LINE('',#20223,#4632);
#3468=LINE('',#20225,#4633);
#3469=LINE('',#20226,#4634);
#3470=LINE('',#20229,#4635);
#3471=LINE('',#20231,#4636);
#3472=LINE('',#20232,#4637);
#3473=LINE('',#20235,#4638);
#3474=LINE('',#20237,#4639);
#3475=LINE('',#20238,#4640);
#3476=LINE('',#20241,#4641);
#3477=LINE('',#20243,#4642);
#3478=LINE('',#20244,#4643);
#3479=LINE('',#20247,#4644);
#3480=LINE('',#20249,#4645);
#3481=LINE('',#20250,#4646);
#3482=LINE('',#20253,#4647);
#3483=LINE('',#20255,#4648);
#3484=LINE('',#20256,#4649);
#3485=LINE('',#20259,#4650);
#3486=LINE('',#20261,#4651);
#3487=LINE('',#20262,#4652);
#3488=LINE('',#20265,#4653);
#3489=LINE('',#20267,#4654);
#3490=LINE('',#20268,#4655);
#3491=LINE('',#20271,#4656);
#3492=LINE('',#20273,#4657);
#3493=LINE('',#20274,#4658);
#3494=LINE('',#20277,#4659);
#3495=LINE('',#20279,#4660);
#3496=LINE('',#20280,#4661);
#3497=LINE('',#20283,#4662);
#3498=LINE('',#20285,#4663);
#3499=LINE('',#20286,#4664);
#3500=LINE('',#20289,#4665);
#3501=LINE('',#20291,#4666);
#3502=LINE('',#20292,#4667);
#3503=LINE('',#20295,#4668);
#3504=LINE('',#20297,#4669);
#3505=LINE('',#20298,#4670);
#3506=LINE('',#20301,#4671);
#3507=LINE('',#20303,#4672);
#3508=LINE('',#20304,#4673);
#3509=LINE('',#20307,#4674);
#3510=LINE('',#20309,#4675);
#3511=LINE('',#20310,#4676);
#3512=LINE('',#20313,#4677);
#3513=LINE('',#20315,#4678);
#3514=LINE('',#20316,#4679);
#3515=LINE('',#20319,#4680);
#3516=LINE('',#20321,#4681);
#3517=LINE('',#20322,#4682);
#3518=LINE('',#20325,#4683);
#3519=LINE('',#20327,#4684);
#3520=LINE('',#20328,#4685);
#3521=LINE('',#20331,#4686);
#3522=LINE('',#20333,#4687);
#3523=LINE('',#20334,#4688);
#3524=LINE('',#20337,#4689);
#3525=LINE('',#20339,#4690);
#3526=LINE('',#20340,#4691);
#3527=LINE('',#20343,#4692);
#3528=LINE('',#20345,#4693);
#3529=LINE('',#20346,#4694);
#3530=LINE('',#20349,#4695);
#3531=LINE('',#20351,#4696);
#3532=LINE('',#20352,#4697);
#3533=LINE('',#20355,#4698);
#3534=LINE('',#20357,#4699);
#3535=LINE('',#20358,#4700);
#3536=LINE('',#20361,#4701);
#3537=LINE('',#20363,#4702);
#3538=LINE('',#20364,#4703);
#3539=LINE('',#20367,#4704);
#3540=LINE('',#20369,#4705);
#3541=LINE('',#20370,#4706);
#3542=LINE('',#20373,#4707);
#3543=LINE('',#20375,#4708);
#3544=LINE('',#20376,#4709);
#3545=LINE('',#20379,#4710);
#3546=LINE('',#20381,#4711);
#3547=LINE('',#20382,#4712);
#3548=LINE('',#20385,#4713);
#3549=LINE('',#20387,#4714);
#3550=LINE('',#20388,#4715);
#3551=LINE('',#20391,#4716);
#3552=LINE('',#20393,#4717);
#3553=LINE('',#20394,#4718);
#3554=LINE('',#20397,#4719);
#3555=LINE('',#20399,#4720);
#3556=LINE('',#20400,#4721);
#3557=LINE('',#20403,#4722);
#3558=LINE('',#20405,#4723);
#3559=LINE('',#20406,#4724);
#3560=LINE('',#20409,#4725);
#3561=LINE('',#20411,#4726);
#3562=LINE('',#20412,#4727);
#3563=LINE('',#20415,#4728);
#3564=LINE('',#20417,#4729);
#3565=LINE('',#20418,#4730);
#3566=LINE('',#20421,#4731);
#3567=LINE('',#20423,#4732);
#3568=LINE('',#20424,#4733);
#3569=LINE('',#20427,#4734);
#3570=LINE('',#20429,#4735);
#3571=LINE('',#20430,#4736);
#3572=LINE('',#20433,#4737);
#3573=LINE('',#20435,#4738);
#3574=LINE('',#20436,#4739);
#3575=LINE('',#20439,#4740);
#3576=LINE('',#20441,#4741);
#3577=LINE('',#20442,#4742);
#3578=LINE('',#20445,#4743);
#3579=LINE('',#20447,#4744);
#3580=LINE('',#20448,#4745);
#3581=LINE('',#20451,#4746);
#3582=LINE('',#20453,#4747);
#3583=LINE('',#20454,#4748);
#3584=LINE('',#20457,#4749);
#3585=LINE('',#20459,#4750);
#3586=LINE('',#20460,#4751);
#3587=LINE('',#20463,#4752);
#3588=LINE('',#20465,#4753);
#3589=LINE('',#20466,#4754);
#3590=LINE('',#20469,#4755);
#3591=LINE('',#20471,#4756);
#3592=LINE('',#20472,#4757);
#3593=LINE('',#20475,#4758);
#3594=LINE('',#20477,#4759);
#3595=LINE('',#20478,#4760);
#3596=LINE('',#20481,#4761);
#3597=LINE('',#20483,#4762);
#3598=LINE('',#20484,#4763);
#3599=LINE('',#20487,#4764);
#3600=LINE('',#20489,#4765);
#3601=LINE('',#20490,#4766);
#3602=LINE('',#20493,#4767);
#3603=LINE('',#20495,#4768);
#3604=LINE('',#20496,#4769);
#3605=LINE('',#20499,#4770);
#3606=LINE('',#20501,#4771);
#3607=LINE('',#20502,#4772);
#3608=LINE('',#20505,#4773);
#3609=LINE('',#20507,#4774);
#3610=LINE('',#20508,#4775);
#3611=LINE('',#20511,#4776);
#3612=LINE('',#20513,#4777);
#3613=LINE('',#20514,#4778);
#3614=LINE('',#20517,#4779);
#3615=LINE('',#20519,#4780);
#3616=LINE('',#20520,#4781);
#3617=LINE('',#20523,#4782);
#3618=LINE('',#20525,#4783);
#3619=LINE('',#20526,#4784);
#3620=LINE('',#20529,#4785);
#3621=LINE('',#20531,#4786);
#3622=LINE('',#20532,#4787);
#3623=LINE('',#20535,#4788);
#3624=LINE('',#20537,#4789);
#3625=LINE('',#20538,#4790);
#3626=LINE('',#20541,#4791);
#3627=LINE('',#20543,#4792);
#3628=LINE('',#20544,#4793);
#3629=LINE('',#20547,#4794);
#3630=LINE('',#20549,#4795);
#3631=LINE('',#20550,#4796);
#3632=LINE('',#20553,#4797);
#3633=LINE('',#20555,#4798);
#3634=LINE('',#20556,#4799);
#3635=LINE('',#20559,#4800);
#3636=LINE('',#20561,#4801);
#3637=LINE('',#20562,#4802);
#3638=LINE('',#20565,#4803);
#3639=LINE('',#20567,#4804);
#3640=LINE('',#20568,#4805);
#3641=LINE('',#20571,#4806);
#3642=LINE('',#20573,#4807);
#3643=LINE('',#20574,#4808);
#3644=LINE('',#20577,#4809);
#3645=LINE('',#20579,#4810);
#3646=LINE('',#20580,#4811);
#3647=LINE('',#20583,#4812);
#3648=LINE('',#20585,#4813);
#3649=LINE('',#20586,#4814);
#3650=LINE('',#20589,#4815);
#3651=LINE('',#20591,#4816);
#3652=LINE('',#20592,#4817);
#3653=LINE('',#20595,#4818);
#3654=LINE('',#20597,#4819);
#3655=LINE('',#20598,#4820);
#3656=LINE('',#20601,#4821);
#3657=LINE('',#20603,#4822);
#3658=LINE('',#20604,#4823);
#3659=LINE('',#20607,#4824);
#3660=LINE('',#20609,#4825);
#3661=LINE('',#20610,#4826);
#3662=LINE('',#20613,#4827);
#3663=LINE('',#20615,#4828);
#3664=LINE('',#20616,#4829);
#3665=LINE('',#20619,#4830);
#3666=LINE('',#20621,#4831);
#3667=LINE('',#20622,#4832);
#3668=LINE('',#20625,#4833);
#3669=LINE('',#20627,#4834);
#3670=LINE('',#20628,#4835);
#3671=LINE('',#20631,#4836);
#3672=LINE('',#20633,#4837);
#3673=LINE('',#20634,#4838);
#3674=LINE('',#20637,#4839);
#3675=LINE('',#20639,#4840);
#3676=LINE('',#20640,#4841);
#3677=LINE('',#20643,#4842);
#3678=LINE('',#20645,#4843);
#3679=LINE('',#20646,#4844);
#3680=LINE('',#20649,#4845);
#3681=LINE('',#20651,#4846);
#3682=LINE('',#20652,#4847);
#3683=LINE('',#20655,#4848);
#3684=LINE('',#20657,#4849);
#3685=LINE('',#20658,#4850);
#3686=LINE('',#20661,#4851);
#3687=LINE('',#20663,#4852);
#3688=LINE('',#20664,#4853);
#3689=LINE('',#20667,#4854);
#3690=LINE('',#20669,#4855);
#3691=LINE('',#20670,#4856);
#3692=LINE('',#20673,#4857);
#3693=LINE('',#20675,#4858);
#3694=LINE('',#20676,#4859);
#3695=LINE('',#20679,#4860);
#3696=LINE('',#20681,#4861);
#3697=LINE('',#20682,#4862);
#3698=LINE('',#20685,#4863);
#3699=LINE('',#20687,#4864);
#3700=LINE('',#20688,#4865);
#3701=LINE('',#20691,#4866);
#3702=LINE('',#20693,#4867);
#3703=LINE('',#20694,#4868);
#3704=LINE('',#20697,#4869);
#3705=LINE('',#20699,#4870);
#3706=LINE('',#20700,#4871);
#3707=LINE('',#20703,#4872);
#3708=LINE('',#20705,#4873);
#3709=LINE('',#20706,#4874);
#3710=LINE('',#20709,#4875);
#3711=LINE('',#20711,#4876);
#3712=LINE('',#20712,#4877);
#3713=LINE('',#20715,#4878);
#3714=LINE('',#20717,#4879);
#3715=LINE('',#20718,#4880);
#3716=LINE('',#20721,#4881);
#3717=LINE('',#20723,#4882);
#3718=LINE('',#20724,#4883);
#3719=LINE('',#20727,#4884);
#3720=LINE('',#20729,#4885);
#3721=LINE('',#20730,#4886);
#3722=LINE('',#20733,#4887);
#3723=LINE('',#20735,#4888);
#3724=LINE('',#20736,#4889);
#3725=LINE('',#20739,#4890);
#3726=LINE('',#20741,#4891);
#3727=LINE('',#20742,#4892);
#3728=LINE('',#20745,#4893);
#3729=LINE('',#20747,#4894);
#3730=LINE('',#20748,#4895);
#3731=LINE('',#20751,#4896);
#3732=LINE('',#20753,#4897);
#3733=LINE('',#20754,#4898);
#3734=LINE('',#20757,#4899);
#3735=LINE('',#20759,#4900);
#3736=LINE('',#20760,#4901);
#3737=LINE('',#20762,#4902);
#3738=LINE('',#20763,#4903);
#3739=LINE('',#20769,#4904);
#3740=LINE('',#20771,#4905);
#4407=VECTOR('',#15867,0.425);
#4408=VECTOR('',#15874,1.);
#4409=VECTOR('',#15875,1.);
#4410=VECTOR('',#15876,1.);
#4411=VECTOR('',#15877,1.);
#4412=VECTOR('',#15880,1.);
#4413=VECTOR('',#15881,1.);
#4414=VECTOR('',#15882,1.);
#4415=VECTOR('',#15883,1.);
#4416=VECTOR('',#15888,1.);
#4417=VECTOR('',#15889,1.);
#4418=VECTOR('',#15890,1.);
#4419=VECTOR('',#15897,1.);
#4420=VECTOR('',#15898,1.);
#4421=VECTOR('',#15899,1.);
#4422=VECTOR('',#15904,1.);
#4423=VECTOR('',#15905,1.);
#4424=VECTOR('',#15906,1.);
#4425=VECTOR('',#15909,1.);
#4426=VECTOR('',#15910,1.);
#4427=VECTOR('',#15911,1.);
#4428=VECTOR('',#15914,1.);
#4429=VECTOR('',#15915,1.);
#4430=VECTOR('',#15916,1.);
#4431=VECTOR('',#15919,1.);
#4432=VECTOR('',#15920,1.);
#4433=VECTOR('',#15921,1.);
#4434=VECTOR('',#15924,1.);
#4435=VECTOR('',#15925,1.);
#4436=VECTOR('',#15926,1.);
#4437=VECTOR('',#15929,1.);
#4438=VECTOR('',#15930,1.);
#4439=VECTOR('',#15931,1.);
#4440=VECTOR('',#15934,1.);
#4441=VECTOR('',#15935,1.);
#4442=VECTOR('',#15936,1.);
#4443=VECTOR('',#15939,1.);
#4444=VECTOR('',#15940,1.);
#4445=VECTOR('',#15941,1.);
#4446=VECTOR('',#15944,1.);
#4447=VECTOR('',#15945,1.);
#4448=VECTOR('',#15946,1.);
#4449=VECTOR('',#15949,1.);
#4450=VECTOR('',#15950,1.);
#4451=VECTOR('',#15951,1.);
#4452=VECTOR('',#15954,1.);
#4453=VECTOR('',#15955,1.);
#4454=VECTOR('',#15956,1.);
#4455=VECTOR('',#15959,1.);
#4456=VECTOR('',#15960,1.);
#4457=VECTOR('',#15961,1.);
#4458=VECTOR('',#15964,1.);
#4459=VECTOR('',#15965,1.);
#4460=VECTOR('',#15966,1.);
#4461=VECTOR('',#15969,1.);
#4462=VECTOR('',#15970,1.);
#4463=VECTOR('',#15971,1.);
#4464=VECTOR('',#15974,1.);
#4465=VECTOR('',#15975,1.);
#4466=VECTOR('',#15976,1.);
#4467=VECTOR('',#15979,1.);
#4468=VECTOR('',#15980,1.);
#4469=VECTOR('',#15981,1.);
#4470=VECTOR('',#15984,1.);
#4471=VECTOR('',#15985,1.);
#4472=VECTOR('',#15986,1.);
#4473=VECTOR('',#15989,1.);
#4474=VECTOR('',#15990,1.);
#4475=VECTOR('',#15991,1.);
#4476=VECTOR('',#15994,1.);
#4477=VECTOR('',#15995,1.);
#4478=VECTOR('',#15996,1.);
#4479=VECTOR('',#15999,1.);
#4480=VECTOR('',#16000,1.);
#4481=VECTOR('',#16001,1.);
#4482=VECTOR('',#16004,1.);
#4483=VECTOR('',#16005,1.);
#4484=VECTOR('',#16006,1.);
#4485=VECTOR('',#16009,1.);
#4486=VECTOR('',#16010,1.);
#4487=VECTOR('',#16011,1.);
#4488=VECTOR('',#16014,1.);
#4489=VECTOR('',#16015,1.);
#4490=VECTOR('',#16016,1.);
#4491=VECTOR('',#16019,1.);
#4492=VECTOR('',#16020,1.);
#4493=VECTOR('',#16021,1.);
#4494=VECTOR('',#16024,1.);
#4495=VECTOR('',#16025,1.);
#4496=VECTOR('',#16026,1.);
#4497=VECTOR('',#16029,1.);
#4498=VECTOR('',#16030,1.);
#4499=VECTOR('',#16031,1.);
#4500=VECTOR('',#16034,1.);
#4501=VECTOR('',#16035,1.);
#4502=VECTOR('',#16036,1.);
#4503=VECTOR('',#16039,1.);
#4504=VECTOR('',#16040,1.);
#4505=VECTOR('',#16041,1.);
#4506=VECTOR('',#16044,1.);
#4507=VECTOR('',#16045,1.);
#4508=VECTOR('',#16046,1.);
#4509=VECTOR('',#16049,1.);
#4510=VECTOR('',#16050,1.);
#4511=VECTOR('',#16051,1.);
#4512=VECTOR('',#16054,1.);
#4513=VECTOR('',#16055,1.);
#4514=VECTOR('',#16056,1.);
#4515=VECTOR('',#16059,1.);
#4516=VECTOR('',#16060,1.);
#4517=VECTOR('',#16061,1.);
#4518=VECTOR('',#16064,1.);
#4519=VECTOR('',#16065,1.);
#4520=VECTOR('',#16066,1.);
#4521=VECTOR('',#16069,1.);
#4522=VECTOR('',#16070,1.);
#4523=VECTOR('',#16071,1.);
#4524=VECTOR('',#16074,1.);
#4525=VECTOR('',#16075,1.);
#4526=VECTOR('',#16076,1.);
#4527=VECTOR('',#16079,1.);
#4528=VECTOR('',#16080,1.);
#4529=VECTOR('',#16081,1.);
#4530=VECTOR('',#16084,1.);
#4531=VECTOR('',#16085,1.);
#4532=VECTOR('',#16086,1.);
#4533=VECTOR('',#16089,1.);
#4534=VECTOR('',#16090,1.);
#4535=VECTOR('',#16091,1.);
#4536=VECTOR('',#16094,1.);
#4537=VECTOR('',#16095,1.);
#4538=VECTOR('',#16096,1.);
#4539=VECTOR('',#16099,1.);
#4540=VECTOR('',#16100,1.);
#4541=VECTOR('',#16101,1.);
#4542=VECTOR('',#16104,1.);
#4543=VECTOR('',#16105,1.);
#4544=VECTOR('',#16106,1.);
#4545=VECTOR('',#16109,1.);
#4546=VECTOR('',#16110,1.);
#4547=VECTOR('',#16111,1.);
#4548=VECTOR('',#16114,1.);
#4549=VECTOR('',#16115,1.);
#4550=VECTOR('',#16116,1.);
#4551=VECTOR('',#16119,1.);
#4552=VECTOR('',#16120,1.);
#4553=VECTOR('',#16121,1.);
#4554=VECTOR('',#16124,1.);
#4555=VECTOR('',#16125,1.);
#4556=VECTOR('',#16126,1.);
#4557=VECTOR('',#16129,1.);
#4558=VECTOR('',#16130,1.);
#4559=VECTOR('',#16131,1.);
#4560=VECTOR('',#16134,1.);
#4561=VECTOR('',#16135,1.);
#4562=VECTOR('',#16136,1.);
#4563=VECTOR('',#16139,1.);
#4564=VECTOR('',#16140,1.);
#4565=VECTOR('',#16141,1.);
#4566=VECTOR('',#16144,1.);
#4567=VECTOR('',#16145,1.);
#4568=VECTOR('',#16146,1.);
#4569=VECTOR('',#16149,1.);
#4570=VECTOR('',#16150,1.);
#4571=VECTOR('',#16151,1.);
#4572=VECTOR('',#16154,1.);
#4573=VECTOR('',#16155,1.);
#4574=VECTOR('',#16156,1.);
#4575=VECTOR('',#16159,1.);
#4576=VECTOR('',#16160,1.);
#4577=VECTOR('',#16161,1.);
#4578=VECTOR('',#16164,1.);
#4579=VECTOR('',#16165,1.);
#4580=VECTOR('',#16166,1.);
#4581=VECTOR('',#16169,1.);
#4582=VECTOR('',#16170,1.);
#4583=VECTOR('',#16171,1.);
#4584=VECTOR('',#16174,1.);
#4585=VECTOR('',#16175,1.);
#4586=VECTOR('',#16176,1.);
#4587=VECTOR('',#16179,1.);
#4588=VECTOR('',#16180,1.);
#4589=VECTOR('',#16181,1.);
#4590=VECTOR('',#16184,1.);
#4591=VECTOR('',#16185,1.);
#4592=VECTOR('',#16186,1.);
#4593=VECTOR('',#16189,1.);
#4594=VECTOR('',#16190,1.);
#4595=VECTOR('',#16191,1.);
#4596=VECTOR('',#16194,1.);
#4597=VECTOR('',#16195,1.);
#4598=VECTOR('',#16196,1.);
#4599=VECTOR('',#16199,1.);
#4600=VECTOR('',#16200,1.);
#4601=VECTOR('',#16201,1.);
#4602=VECTOR('',#16204,1.);
#4603=VECTOR('',#16205,1.);
#4604=VECTOR('',#16206,1.);
#4605=VECTOR('',#16209,1.);
#4606=VECTOR('',#16210,1.);
#4607=VECTOR('',#16211,1.);
#4608=VECTOR('',#16214,1.);
#4609=VECTOR('',#16215,1.);
#4610=VECTOR('',#16216,1.);
#4611=VECTOR('',#16219,1.);
#4612=VECTOR('',#16220,1.);
#4613=VECTOR('',#16221,1.);
#4614=VECTOR('',#16224,1.);
#4615=VECTOR('',#16225,1.);
#4616=VECTOR('',#16226,1.);
#4617=VECTOR('',#16229,1.);
#4618=VECTOR('',#16230,1.);
#4619=VECTOR('',#16231,1.);
#4620=VECTOR('',#16234,1.);
#4621=VECTOR('',#16235,1.);
#4622=VECTOR('',#16236,1.);
#4623=VECTOR('',#16239,1.);
#4624=VECTOR('',#16240,1.);
#4625=VECTOR('',#16241,1.);
#4626=VECTOR('',#16244,1.);
#4627=VECTOR('',#16245,1.);
#4628=VECTOR('',#16246,1.);
#4629=VECTOR('',#16249,1.);
#4630=VECTOR('',#16250,1.);
#4631=VECTOR('',#16251,1.);
#4632=VECTOR('',#16254,1.);
#4633=VECTOR('',#16255,1.);
#4634=VECTOR('',#16256,1.);
#4635=VECTOR('',#16259,1.);
#4636=VECTOR('',#16260,1.);
#4637=VECTOR('',#16261,1.);
#4638=VECTOR('',#16264,1.);
#4639=VECTOR('',#16265,1.);
#4640=VECTOR('',#16266,1.);
#4641=VECTOR('',#16269,1.);
#4642=VECTOR('',#16270,1.);
#4643=VECTOR('',#16271,1.);
#4644=VECTOR('',#16274,1.);
#4645=VECTOR('',#16275,1.);
#4646=VECTOR('',#16276,1.);
#4647=VECTOR('',#16279,1.);
#4648=VECTOR('',#16280,1.);
#4649=VECTOR('',#16281,1.);
#4650=VECTOR('',#16284,1.);
#4651=VECTOR('',#16285,1.);
#4652=VECTOR('',#16286,1.);
#4653=VECTOR('',#16289,1.);
#4654=VECTOR('',#16290,1.);
#4655=VECTOR('',#16291,1.);
#4656=VECTOR('',#16294,1.);
#4657=VECTOR('',#16295,1.);
#4658=VECTOR('',#16296,1.);
#4659=VECTOR('',#16299,1.);
#4660=VECTOR('',#16300,1.);
#4661=VECTOR('',#16301,1.);
#4662=VECTOR('',#16304,1.);
#4663=VECTOR('',#16305,1.);
#4664=VECTOR('',#16306,1.);
#4665=VECTOR('',#16309,1.);
#4666=VECTOR('',#16310,1.);
#4667=VECTOR('',#16311,1.);
#4668=VECTOR('',#16314,1.);
#4669=VECTOR('',#16315,1.);
#4670=VECTOR('',#16316,1.);
#4671=VECTOR('',#16319,1.);
#4672=VECTOR('',#16320,1.);
#4673=VECTOR('',#16321,1.);
#4674=VECTOR('',#16324,1.);
#4675=VECTOR('',#16325,1.);
#4676=VECTOR('',#16326,1.);
#4677=VECTOR('',#16329,1.);
#4678=VECTOR('',#16330,1.);
#4679=VECTOR('',#16331,1.);
#4680=VECTOR('',#16334,1.);
#4681=VECTOR('',#16335,1.);
#4682=VECTOR('',#16336,1.);
#4683=VECTOR('',#16339,1.);
#4684=VECTOR('',#16340,1.);
#4685=VECTOR('',#16341,1.);
#4686=VECTOR('',#16344,1.);
#4687=VECTOR('',#16345,1.);
#4688=VECTOR('',#16346,1.);
#4689=VECTOR('',#16349,1.);
#4690=VECTOR('',#16350,1.);
#4691=VECTOR('',#16351,1.);
#4692=VECTOR('',#16354,1.);
#4693=VECTOR('',#16355,1.);
#4694=VECTOR('',#16356,1.);
#4695=VECTOR('',#16359,1.);
#4696=VECTOR('',#16360,1.);
#4697=VECTOR('',#16361,1.);
#4698=VECTOR('',#16364,1.);
#4699=VECTOR('',#16365,1.);
#4700=VECTOR('',#16366,1.);
#4701=VECTOR('',#16369,1.);
#4702=VECTOR('',#16370,1.);
#4703=VECTOR('',#16371,1.);
#4704=VECTOR('',#16374,1.);
#4705=VECTOR('',#16375,1.);
#4706=VECTOR('',#16376,1.);
#4707=VECTOR('',#16379,1.);
#4708=VECTOR('',#16380,1.);
#4709=VECTOR('',#16381,1.);
#4710=VECTOR('',#16384,1.);
#4711=VECTOR('',#16385,1.);
#4712=VECTOR('',#16386,1.);
#4713=VECTOR('',#16389,1.);
#4714=VECTOR('',#16390,1.);
#4715=VECTOR('',#16391,1.);
#4716=VECTOR('',#16394,1.);
#4717=VECTOR('',#16395,1.);
#4718=VECTOR('',#16396,1.);
#4719=VECTOR('',#16399,1.);
#4720=VECTOR('',#16400,1.);
#4721=VECTOR('',#16401,1.);
#4722=VECTOR('',#16404,1.);
#4723=VECTOR('',#16405,1.);
#4724=VECTOR('',#16406,1.);
#4725=VECTOR('',#16409,1.);
#4726=VECTOR('',#16410,1.);
#4727=VECTOR('',#16411,1.);
#4728=VECTOR('',#16414,1.);
#4729=VECTOR('',#16415,1.);
#4730=VECTOR('',#16416,1.);
#4731=VECTOR('',#16419,1.);
#4732=VECTOR('',#16420,1.);
#4733=VECTOR('',#16421,1.);
#4734=VECTOR('',#16424,1.);
#4735=VECTOR('',#16425,1.);
#4736=VECTOR('',#16426,1.);
#4737=VECTOR('',#16429,1.);
#4738=VECTOR('',#16430,1.);
#4739=VECTOR('',#16431,1.);
#4740=VECTOR('',#16434,1.);
#4741=VECTOR('',#16435,1.);
#4742=VECTOR('',#16436,1.);
#4743=VECTOR('',#16439,1.);
#4744=VECTOR('',#16440,1.);
#4745=VECTOR('',#16441,1.);
#4746=VECTOR('',#16444,1.);
#4747=VECTOR('',#16445,1.);
#4748=VECTOR('',#16446,1.);
#4749=VECTOR('',#16449,1.);
#4750=VECTOR('',#16450,1.);
#4751=VECTOR('',#16451,1.);
#4752=VECTOR('',#16454,1.);
#4753=VECTOR('',#16455,1.);
#4754=VECTOR('',#16456,1.);
#4755=VECTOR('',#16459,1.);
#4756=VECTOR('',#16460,1.);
#4757=VECTOR('',#16461,1.);
#4758=VECTOR('',#16464,1.);
#4759=VECTOR('',#16465,1.);
#4760=VECTOR('',#16466,1.);
#4761=VECTOR('',#16469,1.);
#4762=VECTOR('',#16470,1.);
#4763=VECTOR('',#16471,1.);
#4764=VECTOR('',#16474,1.);
#4765=VECTOR('',#16475,1.);
#4766=VECTOR('',#16476,1.);
#4767=VECTOR('',#16479,1.);
#4768=VECTOR('',#16480,1.);
#4769=VECTOR('',#16481,1.);
#4770=VECTOR('',#16484,1.);
#4771=VECTOR('',#16485,1.);
#4772=VECTOR('',#16486,1.);
#4773=VECTOR('',#16489,1.);
#4774=VECTOR('',#16490,1.);
#4775=VECTOR('',#16491,1.);
#4776=VECTOR('',#16494,1.);
#4777=VECTOR('',#16495,1.);
#4778=VECTOR('',#16496,1.);
#4779=VECTOR('',#16499,1.);
#4780=VECTOR('',#16500,1.);
#4781=VECTOR('',#16501,1.);
#4782=VECTOR('',#16504,1.);
#4783=VECTOR('',#16505,1.);
#4784=VECTOR('',#16506,1.);
#4785=VECTOR('',#16509,1.);
#4786=VECTOR('',#16510,1.);
#4787=VECTOR('',#16511,1.);
#4788=VECTOR('',#16514,1.);
#4789=VECTOR('',#16515,1.);
#4790=VECTOR('',#16516,1.);
#4791=VECTOR('',#16519,1.);
#4792=VECTOR('',#16520,1.);
#4793=VECTOR('',#16521,1.);
#4794=VECTOR('',#16524,1.);
#4795=VECTOR('',#16525,1.);
#4796=VECTOR('',#16526,1.);
#4797=VECTOR('',#16529,1.);
#4798=VECTOR('',#16530,1.);
#4799=VECTOR('',#16531,1.);
#4800=VECTOR('',#16534,1.);
#4801=VECTOR('',#16535,1.);
#4802=VECTOR('',#16536,1.);
#4803=VECTOR('',#16539,1.);
#4804=VECTOR('',#16540,1.);
#4805=VECTOR('',#16541,1.);
#4806=VECTOR('',#16544,1.);
#4807=VECTOR('',#16545,1.);
#4808=VECTOR('',#16546,1.);
#4809=VECTOR('',#16549,1.);
#4810=VECTOR('',#16550,1.);
#4811=VECTOR('',#16551,1.);
#4812=VECTOR('',#16554,1.);
#4813=VECTOR('',#16555,1.);
#4814=VECTOR('',#16556,1.);
#4815=VECTOR('',#16559,1.);
#4816=VECTOR('',#16560,1.);
#4817=VECTOR('',#16561,1.);
#4818=VECTOR('',#16564,1.);
#4819=VECTOR('',#16565,1.);
#4820=VECTOR('',#16566,1.);
#4821=VECTOR('',#16569,1.);
#4822=VECTOR('',#16570,1.);
#4823=VECTOR('',#16571,1.);
#4824=VECTOR('',#16574,1.);
#4825=VECTOR('',#16575,1.);
#4826=VECTOR('',#16576,1.);
#4827=VECTOR('',#16579,1.);
#4828=VECTOR('',#16580,1.);
#4829=VECTOR('',#16581,1.);
#4830=VECTOR('',#16584,1.);
#4831=VECTOR('',#16585,1.);
#4832=VECTOR('',#16586,1.);
#4833=VECTOR('',#16589,1.);
#4834=VECTOR('',#16590,1.);
#4835=VECTOR('',#16591,1.);
#4836=VECTOR('',#16594,1.);
#4837=VECTOR('',#16595,1.);
#4838=VECTOR('',#16596,1.);
#4839=VECTOR('',#16599,1.);
#4840=VECTOR('',#16600,1.);
#4841=VECTOR('',#16601,1.);
#4842=VECTOR('',#16604,1.);
#4843=VECTOR('',#16605,1.);
#4844=VECTOR('',#16606,1.);
#4845=VECTOR('',#16609,1.);
#4846=VECTOR('',#16610,1.);
#4847=VECTOR('',#16611,1.);
#4848=VECTOR('',#16614,1.);
#4849=VECTOR('',#16615,1.);
#4850=VECTOR('',#16616,1.);
#4851=VECTOR('',#16619,1.);
#4852=VECTOR('',#16620,1.);
#4853=VECTOR('',#16621,1.);
#4854=VECTOR('',#16624,1.);
#4855=VECTOR('',#16625,1.);
#4856=VECTOR('',#16626,1.);
#4857=VECTOR('',#16629,1.);
#4858=VECTOR('',#16630,1.);
#4859=VECTOR('',#16631,1.);
#4860=VECTOR('',#16634,1.);
#4861=VECTOR('',#16635,1.);
#4862=VECTOR('',#16636,1.);
#4863=VECTOR('',#16639,1.);
#4864=VECTOR('',#16640,1.);
#4865=VECTOR('',#16641,1.);
#4866=VECTOR('',#16644,1.);
#4867=VECTOR('',#16645,1.);
#4868=VECTOR('',#16646,1.);
#4869=VECTOR('',#16649,1.);
#4870=VECTOR('',#16650,1.);
#4871=VECTOR('',#16651,1.);
#4872=VECTOR('',#16654,1.);
#4873=VECTOR('',#16655,1.);
#4874=VECTOR('',#16656,1.);
#4875=VECTOR('',#16659,1.);
#4876=VECTOR('',#16660,1.);
#4877=VECTOR('',#16661,1.);
#4878=VECTOR('',#16664,1.);
#4879=VECTOR('',#16665,1.);
#4880=VECTOR('',#16666,1.);
#4881=VECTOR('',#16669,1.);
#4882=VECTOR('',#16670,1.);
#4883=VECTOR('',#16671,1.);
#4884=VECTOR('',#16674,1.);
#4885=VECTOR('',#16675,1.);
#4886=VECTOR('',#16676,1.);
#4887=VECTOR('',#16679,1.);
#4888=VECTOR('',#16680,1.);
#4889=VECTOR('',#16681,1.);
#4890=VECTOR('',#16684,1.);
#4891=VECTOR('',#16685,1.);
#4892=VECTOR('',#16686,1.);
#4893=VECTOR('',#16689,1.);
#4894=VECTOR('',#16690,1.);
#4895=VECTOR('',#16691,1.);
#4896=VECTOR('',#16694,1.);
#4897=VECTOR('',#16695,1.);
#4898=VECTOR('',#16696,1.);
#4899=VECTOR('',#16699,1.);
#4900=VECTOR('',#16700,1.);
#4901=VECTOR('',#16701,1.);
#4902=VECTOR('',#16704,1.);
#4903=VECTOR('',#16705,1.);
#4904=VECTOR('',#16714,1.);
#4905=VECTOR('',#16715,1.);
#5469=CIRCLE('',#13758,0.425);
#5470=CIRCLE('',#13759,0.425);
#5471=CIRCLE('',#13764,1.);
#5472=CIRCLE('',#13765,1.);
#5473=CIRCLE('',#13767,1.);
#5474=CIRCLE('',#13768,1.);
#5475=CIRCLE('',#13933,1.);
#5476=CIRCLE('',#13934,1.);
#6048=VERTEX_POINT('',#19759);
#6049=VERTEX_POINT('',#19761);
#6050=VERTEX_POINT('',#19766);
#6051=VERTEX_POINT('',#19767);
#6052=VERTEX_POINT('',#19769);
#6053=VERTEX_POINT('',#19771);
#6054=VERTEX_POINT('',#19775);
#6055=VERTEX_POINT('',#19776);
#6056=VERTEX_POINT('',#19778);
#6057=VERTEX_POINT('',#19780);
#6058=VERTEX_POINT('',#19784);
#6059=VERTEX_POINT('',#19786);
#6060=VERTEX_POINT('',#19788);
#6061=VERTEX_POINT('',#19793);
#6062=VERTEX_POINT('',#19795);
#6063=VERTEX_POINT('',#19797);
#6064=VERTEX_POINT('',#19802);
#6065=VERTEX_POINT('',#19804);
#6066=VERTEX_POINT('',#19808);
#6067=VERTEX_POINT('',#19810);
#6068=VERTEX_POINT('',#19814);
#6069=VERTEX_POINT('',#19816);
#6070=VERTEX_POINT('',#19820);
#6071=VERTEX_POINT('',#19822);
#6072=VERTEX_POINT('',#19826);
#6073=VERTEX_POINT('',#19828);
#6074=VERTEX_POINT('',#19832);
#6075=VERTEX_POINT('',#19834);
#6076=VERTEX_POINT('',#19838);
#6077=VERTEX_POINT('',#19840);
#6078=VERTEX_POINT('',#19844);
#6079=VERTEX_POINT('',#19846);
#6080=VERTEX_POINT('',#19850);
#6081=VERTEX_POINT('',#19852);
#6082=VERTEX_POINT('',#19856);
#6083=VERTEX_POINT('',#19858);
#6084=VERTEX_POINT('',#19862);
#6085=VERTEX_POINT('',#19864);
#6086=VERTEX_POINT('',#19868);
#6087=VERTEX_POINT('',#19870);
#6088=VERTEX_POINT('',#19874);
#6089=VERTEX_POINT('',#19876);
#6090=VERTEX_POINT('',#19880);
#6091=VERTEX_POINT('',#19882);
#6092=VERTEX_POINT('',#19886);
#6093=VERTEX_POINT('',#19888);
#6094=VERTEX_POINT('',#19892);
#6095=VERTEX_POINT('',#19894);
#6096=VERTEX_POINT('',#19898);
#6097=VERTEX_POINT('',#19900);
#6098=VERTEX_POINT('',#19904);
#6099=VERTEX_POINT('',#19906);
#6100=VERTEX_POINT('',#19910);
#6101=VERTEX_POINT('',#19912);
#6102=VERTEX_POINT('',#19916);
#6103=VERTEX_POINT('',#19918);
#6104=VERTEX_POINT('',#19922);
#6105=VERTEX_POINT('',#19924);
#6106=VERTEX_POINT('',#19928);
#6107=VERTEX_POINT('',#19930);
#6108=VERTEX_POINT('',#19934);
#6109=VERTEX_POINT('',#19936);
#6110=VERTEX_POINT('',#19940);
#6111=VERTEX_POINT('',#19942);
#6112=VERTEX_POINT('',#19946);
#6113=VERTEX_POINT('',#19948);
#6114=VERTEX_POINT('',#19952);
#6115=VERTEX_POINT('',#19954);
#6116=VERTEX_POINT('',#19958);
#6117=VERTEX_POINT('',#19960);
#6118=VERTEX_POINT('',#19964);
#6119=VERTEX_POINT('',#19966);
#6120=VERTEX_POINT('',#19970);
#6121=VERTEX_POINT('',#19972);
#6122=VERTEX_POINT('',#19976);
#6123=VERTEX_POINT('',#19978);
#6124=VERTEX_POINT('',#19982);
#6125=VERTEX_POINT('',#19984);
#6126=VERTEX_POINT('',#19988);
#6127=VERTEX_POINT('',#19990);
#6128=VERTEX_POINT('',#19994);
#6129=VERTEX_POINT('',#19996);
#6130=VERTEX_POINT('',#20000);
#6131=VERTEX_POINT('',#20002);
#6132=VERTEX_POINT('',#20006);
#6133=VERTEX_POINT('',#20008);
#6134=VERTEX_POINT('',#20012);
#6135=VERTEX_POINT('',#20014);
#6136=VERTEX_POINT('',#20018);
#6137=VERTEX_POINT('',#20020);
#6138=VERTEX_POINT('',#20024);
#6139=VERTEX_POINT('',#20026);
#6140=VERTEX_POINT('',#20030);
#6141=VERTEX_POINT('',#20032);
#6142=VERTEX_POINT('',#20036);
#6143=VERTEX_POINT('',#20038);
#6144=VERTEX_POINT('',#20042);
#6145=VERTEX_POINT('',#20044);
#6146=VERTEX_POINT('',#20048);
#6147=VERTEX_POINT('',#20050);
#6148=VERTEX_POINT('',#20054);
#6149=VERTEX_POINT('',#20056);
#6150=VERTEX_POINT('',#20060);
#6151=VERTEX_POINT('',#20062);
#6152=VERTEX_POINT('',#20066);
#6153=VERTEX_POINT('',#20068);
#6154=VERTEX_POINT('',#20072);
#6155=VERTEX_POINT('',#20074);
#6156=VERTEX_POINT('',#20078);
#6157=VERTEX_POINT('',#20080);
#6158=VERTEX_POINT('',#20084);
#6159=VERTEX_POINT('',#20086);
#6160=VERTEX_POINT('',#20090);
#6161=VERTEX_POINT('',#20092);
#6162=VERTEX_POINT('',#20096);
#6163=VERTEX_POINT('',#20098);
#6164=VERTEX_POINT('',#20102);
#6165=VERTEX_POINT('',#20104);
#6166=VERTEX_POINT('',#20108);
#6167=VERTEX_POINT('',#20110);
#6168=VERTEX_POINT('',#20114);
#6169=VERTEX_POINT('',#20116);
#6170=VERTEX_POINT('',#20120);
#6171=VERTEX_POINT('',#20122);
#6172=VERTEX_POINT('',#20126);
#6173=VERTEX_POINT('',#20128);
#6174=VERTEX_POINT('',#20132);
#6175=VERTEX_POINT('',#20134);
#6176=VERTEX_POINT('',#20138);
#6177=VERTEX_POINT('',#20140);
#6178=VERTEX_POINT('',#20144);
#6179=VERTEX_POINT('',#20146);
#6180=VERTEX_POINT('',#20150);
#6181=VERTEX_POINT('',#20152);
#6182=VERTEX_POINT('',#20156);
#6183=VERTEX_POINT('',#20158);
#6184=VERTEX_POINT('',#20162);
#6185=VERTEX_POINT('',#20164);
#6186=VERTEX_POINT('',#20168);
#6187=VERTEX_POINT('',#20170);
#6188=VERTEX_POINT('',#20174);
#6189=VERTEX_POINT('',#20176);
#6190=VERTEX_POINT('',#20180);
#6191=VERTEX_POINT('',#20182);
#6192=VERTEX_POINT('',#20186);
#6193=VERTEX_POINT('',#20188);
#6194=VERTEX_POINT('',#20192);
#6195=VERTEX_POINT('',#20194);
#6196=VERTEX_POINT('',#20198);
#6197=VERTEX_POINT('',#20200);
#6198=VERTEX_POINT('',#20204);
#6199=VERTEX_POINT('',#20206);
#6200=VERTEX_POINT('',#20210);
#6201=VERTEX_POINT('',#20212);
#6202=VERTEX_POINT('',#20216);
#6203=VERTEX_POINT('',#20218);
#6204=VERTEX_POINT('',#20222);
#6205=VERTEX_POINT('',#20224);
#6206=VERTEX_POINT('',#20228);
#6207=VERTEX_POINT('',#20230);
#6208=VERTEX_POINT('',#20234);
#6209=VERTEX_POINT('',#20236);
#6210=VERTEX_POINT('',#20240);
#6211=VERTEX_POINT('',#20242);
#6212=VERTEX_POINT('',#20246);
#6213=VERTEX_POINT('',#20248);
#6214=VERTEX_POINT('',#20252);
#6215=VERTEX_POINT('',#20254);
#6216=VERTEX_POINT('',#20258);
#6217=VERTEX_POINT('',#20260);
#6218=VERTEX_POINT('',#20264);
#6219=VERTEX_POINT('',#20266);
#6220=VERTEX_POINT('',#20270);
#6221=VERTEX_POINT('',#20272);
#6222=VERTEX_POINT('',#20276);
#6223=VERTEX_POINT('',#20278);
#6224=VERTEX_POINT('',#20282);
#6225=VERTEX_POINT('',#20284);
#6226=VERTEX_POINT('',#20288);
#6227=VERTEX_POINT('',#20290);
#6228=VERTEX_POINT('',#20294);
#6229=VERTEX_POINT('',#20296);
#6230=VERTEX_POINT('',#20300);
#6231=VERTEX_POINT('',#20302);
#6232=VERTEX_POINT('',#20306);
#6233=VERTEX_POINT('',#20308);
#6234=VERTEX_POINT('',#20312);
#6235=VERTEX_POINT('',#20314);
#6236=VERTEX_POINT('',#20318);
#6237=VERTEX_POINT('',#20320);
#6238=VERTEX_POINT('',#20324);
#6239=VERTEX_POINT('',#20326);
#6240=VERTEX_POINT('',#20330);
#6241=VERTEX_POINT('',#20332);
#6242=VERTEX_POINT('',#20336);
#6243=VERTEX_POINT('',#20338);
#6244=VERTEX_POINT('',#20342);
#6245=VERTEX_POINT('',#20344);
#6246=VERTEX_POINT('',#20348);
#6247=VERTEX_POINT('',#20350);
#6248=VERTEX_POINT('',#20354);
#6249=VERTEX_POINT('',#20356);
#6250=VERTEX_POINT('',#20360);
#6251=VERTEX_POINT('',#20362);
#6252=VERTEX_POINT('',#20366);
#6253=VERTEX_POINT('',#20368);
#6254=VERTEX_POINT('',#20372);
#6255=VERTEX_POINT('',#20374);
#6256=VERTEX_POINT('',#20378);
#6257=VERTEX_POINT('',#20380);
#6258=VERTEX_POINT('',#20384);
#6259=VERTEX_POINT('',#20386);
#6260=VERTEX_POINT('',#20390);
#6261=VERTEX_POINT('',#20392);
#6262=VERTEX_POINT('',#20396);
#6263=VERTEX_POINT('',#20398);
#6264=VERTEX_POINT('',#20402);
#6265=VERTEX_POINT('',#20404);
#6266=VERTEX_POINT('',#20408);
#6267=VERTEX_POINT('',#20410);
#6268=VERTEX_POINT('',#20414);
#6269=VERTEX_POINT('',#20416);
#6270=VERTEX_POINT('',#20420);
#6271=VERTEX_POINT('',#20422);
#6272=VERTEX_POINT('',#20426);
#6273=VERTEX_POINT('',#20428);
#6274=VERTEX_POINT('',#20432);
#6275=VERTEX_POINT('',#20434);
#6276=VERTEX_POINT('',#20438);
#6277=VERTEX_POINT('',#20440);
#6278=VERTEX_POINT('',#20444);
#6279=VERTEX_POINT('',#20446);
#6280=VERTEX_POINT('',#20450);
#6281=VERTEX_POINT('',#20452);
#6282=VERTEX_POINT('',#20456);
#6283=VERTEX_POINT('',#20458);
#6284=VERTEX_POINT('',#20462);
#6285=VERTEX_POINT('',#20464);
#6286=VERTEX_POINT('',#20468);
#6287=VERTEX_POINT('',#20470);
#6288=VERTEX_POINT('',#20474);
#6289=VERTEX_POINT('',#20476);
#6290=VERTEX_POINT('',#20480);
#6291=VERTEX_POINT('',#20482);
#6292=VERTEX_POINT('',#20486);
#6293=VERTEX_POINT('',#20488);
#6294=VERTEX_POINT('',#20492);
#6295=VERTEX_POINT('',#20494);
#6296=VERTEX_POINT('',#20498);
#6297=VERTEX_POINT('',#20500);
#6298=VERTEX_POINT('',#20504);
#6299=VERTEX_POINT('',#20506);
#6300=VERTEX_POINT('',#20510);
#6301=VERTEX_POINT('',#20512);
#6302=VERTEX_POINT('',#20516);
#6303=VERTEX_POINT('',#20518);
#6304=VERTEX_POINT('',#20522);
#6305=VERTEX_POINT('',#20524);
#6306=VERTEX_POINT('',#20528);
#6307=VERTEX_POINT('',#20530);
#6308=VERTEX_POINT('',#20534);
#6309=VERTEX_POINT('',#20536);
#6310=VERTEX_POINT('',#20540);
#6311=VERTEX_POINT('',#20542);
#6312=VERTEX_POINT('',#20546);
#6313=VERTEX_POINT('',#20548);
#6314=VERTEX_POINT('',#20552);
#6315=VERTEX_POINT('',#20554);
#6316=VERTEX_POINT('',#20558);
#6317=VERTEX_POINT('',#20560);
#6318=VERTEX_POINT('',#20564);
#6319=VERTEX_POINT('',#20566);
#6320=VERTEX_POINT('',#20570);
#6321=VERTEX_POINT('',#20572);
#6322=VERTEX_POINT('',#20576);
#6323=VERTEX_POINT('',#20578);
#6324=VERTEX_POINT('',#20582);
#6325=VERTEX_POINT('',#20584);
#6326=VERTEX_POINT('',#20588);
#6327=VERTEX_POINT('',#20590);
#6328=VERTEX_POINT('',#20594);
#6329=VERTEX_POINT('',#20596);
#6330=VERTEX_POINT('',#20600);
#6331=VERTEX_POINT('',#20602);
#6332=VERTEX_POINT('',#20606);
#6333=VERTEX_POINT('',#20608);
#6334=VERTEX_POINT('',#20612);
#6335=VERTEX_POINT('',#20614);
#6336=VERTEX_POINT('',#20618);
#6337=VERTEX_POINT('',#20620);
#6338=VERTEX_POINT('',#20624);
#6339=VERTEX_POINT('',#20626);
#6340=VERTEX_POINT('',#20630);
#6341=VERTEX_POINT('',#20632);
#6342=VERTEX_POINT('',#20636);
#6343=VERTEX_POINT('',#20638);
#6344=VERTEX_POINT('',#20642);
#6345=VERTEX_POINT('',#20644);
#6346=VERTEX_POINT('',#20648);
#6347=VERTEX_POINT('',#20650);
#6348=VERTEX_POINT('',#20654);
#6349=VERTEX_POINT('',#20656);
#6350=VERTEX_POINT('',#20660);
#6351=VERTEX_POINT('',#20662);
#6352=VERTEX_POINT('',#20666);
#6353=VERTEX_POINT('',#20668);
#6354=VERTEX_POINT('',#20672);
#6355=VERTEX_POINT('',#20674);
#6356=VERTEX_POINT('',#20678);
#6357=VERTEX_POINT('',#20680);
#6358=VERTEX_POINT('',#20684);
#6359=VERTEX_POINT('',#20686);
#6360=VERTEX_POINT('',#20690);
#6361=VERTEX_POINT('',#20692);
#6362=VERTEX_POINT('',#20696);
#6363=VERTEX_POINT('',#20698);
#6364=VERTEX_POINT('',#20702);
#6365=VERTEX_POINT('',#20704);
#6366=VERTEX_POINT('',#20708);
#6367=VERTEX_POINT('',#20710);
#6368=VERTEX_POINT('',#20714);
#6369=VERTEX_POINT('',#20716);
#6370=VERTEX_POINT('',#20720);
#6371=VERTEX_POINT('',#20722);
#6372=VERTEX_POINT('',#20726);
#6373=VERTEX_POINT('',#20728);
#6374=VERTEX_POINT('',#20732);
#6375=VERTEX_POINT('',#20734);
#6376=VERTEX_POINT('',#20738);
#6377=VERTEX_POINT('',#20740);
#6378=VERTEX_POINT('',#20744);
#6379=VERTEX_POINT('',#20746);
#6380=VERTEX_POINT('',#20750);
#6381=VERTEX_POINT('',#20752);
#6382=VERTEX_POINT('',#20756);
#6383=VERTEX_POINT('',#20758);
#6384=VERTEX_POINT('',#20767);
#6385=VERTEX_POINT('',#20770);
#7381=EDGE_CURVE('',#6048,#6048,#5469,.T.);
#7382=EDGE_CURVE('',#6048,#6049,#3242,.T.);
#7383=EDGE_CURVE('',#6049,#6049,#5470,.T.);
#7384=EDGE_CURVE('',#6050,#6051,#3243,.T.);
#7385=EDGE_CURVE('',#6052,#6050,#3244,.T.);
#7386=EDGE_CURVE('',#6053,#6052,#3245,.T.);
#7387=EDGE_CURVE('',#6053,#6051,#3246,.T.);
#7388=EDGE_CURVE('',#6054,#6055,#3247,.T.);
#7389=EDGE_CURVE('',#6054,#6056,#3248,.T.);
#7390=EDGE_CURVE('',#6057,#6056,#3249,.T.);
#7391=EDGE_CURVE('',#6055,#6057,#3250,.T.);
#7392=EDGE_CURVE('',#6051,#6058,#5471,.T.);
#7393=EDGE_CURVE('',#6059,#6053,#3251,.T.);
#7394=EDGE_CURVE('',#6059,#6060,#3252,.T.);
#7395=EDGE_CURVE('',#6056,#6060,#3253,.T.);
#7396=EDGE_CURVE('',#6058,#6054,#5472,.T.);
#7397=EDGE_CURVE('',#6055,#6061,#5473,.T.);
#7398=EDGE_CURVE('',#6062,#6057,#3254,.T.);
#7399=EDGE_CURVE('',#6063,#6062,#3255,.T.);
#7400=EDGE_CURVE('',#6052,#6063,#3256,.T.);
#7401=EDGE_CURVE('',#6061,#6050,#5474,.T.);
#7402=EDGE_CURVE('',#6063,#6064,#3257,.T.);
#7403=EDGE_CURVE('',#6065,#6062,#3258,.T.);
#7404=EDGE_CURVE('',#6064,#6065,#3259,.T.);
#7405=EDGE_CURVE('',#6064,#6066,#3260,.T.);
#7406=EDGE_CURVE('',#6067,#6065,#3261,.T.);
#7407=EDGE_CURVE('',#6066,#6067,#3262,.T.);
#7408=EDGE_CURVE('',#6066,#6068,#3263,.T.);
#7409=EDGE_CURVE('',#6069,#6067,#3264,.T.);
#7410=EDGE_CURVE('',#6068,#6069,#3265,.T.);
#7411=EDGE_CURVE('',#6068,#6070,#3266,.T.);
#7412=EDGE_CURVE('',#6071,#6069,#3267,.T.);
#7413=EDGE_CURVE('',#6070,#6071,#3268,.T.);
#7414=EDGE_CURVE('',#6070,#6072,#3269,.T.);
#7415=EDGE_CURVE('',#6073,#6071,#3270,.T.);
#7416=EDGE_CURVE('',#6072,#6073,#3271,.T.);
#7417=EDGE_CURVE('',#6072,#6074,#3272,.T.);
#7418=EDGE_CURVE('',#6075,#6073,#3273,.T.);
#7419=EDGE_CURVE('',#6074,#6075,#3274,.T.);
#7420=EDGE_CURVE('',#6074,#6076,#3275,.T.);
#7421=EDGE_CURVE('',#6077,#6075,#3276,.T.);
#7422=EDGE_CURVE('',#6076,#6077,#3277,.T.);
#7423=EDGE_CURVE('',#6076,#6078,#3278,.T.);
#7424=EDGE_CURVE('',#6079,#6077,#3279,.T.);
#7425=EDGE_CURVE('',#6078,#6079,#3280,.T.);
#7426=EDGE_CURVE('',#6078,#6080,#3281,.T.);
#7427=EDGE_CURVE('',#6081,#6079,#3282,.T.);
#7428=EDGE_CURVE('',#6080,#6081,#3283,.T.);
#7429=EDGE_CURVE('',#6080,#6082,#3284,.T.);
#7430=EDGE_CURVE('',#6083,#6081,#3285,.T.);
#7431=EDGE_CURVE('',#6082,#6083,#3286,.T.);
#7432=EDGE_CURVE('',#6082,#6084,#3287,.T.);
#7433=EDGE_CURVE('',#6085,#6083,#3288,.T.);
#7434=EDGE_CURVE('',#6084,#6085,#3289,.T.);
#7435=EDGE_CURVE('',#6084,#6086,#3290,.T.);
#7436=EDGE_CURVE('',#6087,#6085,#3291,.T.);
#7437=EDGE_CURVE('',#6086,#6087,#3292,.T.);
#7438=EDGE_CURVE('',#6086,#6088,#3293,.T.);
#7439=EDGE_CURVE('',#6089,#6087,#3294,.T.);
#7440=EDGE_CURVE('',#6088,#6089,#3295,.T.);
#7441=EDGE_CURVE('',#6088,#6090,#3296,.T.);
#7442=EDGE_CURVE('',#6091,#6089,#3297,.T.);
#7443=EDGE_CURVE('',#6090,#6091,#3298,.T.);
#7444=EDGE_CURVE('',#6090,#6092,#3299,.T.);
#7445=EDGE_CURVE('',#6093,#6091,#3300,.T.);
#7446=EDGE_CURVE('',#6092,#6093,#3301,.T.);
#7447=EDGE_CURVE('',#6092,#6094,#3302,.T.);
#7448=EDGE_CURVE('',#6095,#6093,#3303,.T.);
#7449=EDGE_CURVE('',#6094,#6095,#3304,.T.);
#7450=EDGE_CURVE('',#6094,#6096,#3305,.T.);
#7451=EDGE_CURVE('',#6097,#6095,#3306,.T.);
#7452=EDGE_CURVE('',#6096,#6097,#3307,.T.);
#7453=EDGE_CURVE('',#6096,#6098,#3308,.T.);
#7454=EDGE_CURVE('',#6099,#6097,#3309,.T.);
#7455=EDGE_CURVE('',#6098,#6099,#3310,.T.);
#7456=EDGE_CURVE('',#6098,#6100,#3311,.T.);
#7457=EDGE_CURVE('',#6101,#6099,#3312,.T.);
#7458=EDGE_CURVE('',#6100,#6101,#3313,.T.);
#7459=EDGE_CURVE('',#6100,#6102,#3314,.T.);
#7460=EDGE_CURVE('',#6103,#6101,#3315,.T.);
#7461=EDGE_CURVE('',#6102,#6103,#3316,.T.);
#7462=EDGE_CURVE('',#6102,#6104,#3317,.T.);
#7463=EDGE_CURVE('',#6105,#6103,#3318,.T.);
#7464=EDGE_CURVE('',#6104,#6105,#3319,.T.);
#7465=EDGE_CURVE('',#6104,#6106,#3320,.T.);
#7466=EDGE_CURVE('',#6107,#6105,#3321,.T.);
#7467=EDGE_CURVE('',#6106,#6107,#3322,.T.);
#7468=EDGE_CURVE('',#6106,#6108,#3323,.T.);
#7469=EDGE_CURVE('',#6109,#6107,#3324,.T.);
#7470=EDGE_CURVE('',#6108,#6109,#3325,.T.);
#7471=EDGE_CURVE('',#6108,#6110,#3326,.T.);
#7472=EDGE_CURVE('',#6111,#6109,#3327,.T.);
#7473=EDGE_CURVE('',#6110,#6111,#3328,.T.);
#7474=EDGE_CURVE('',#6110,#6112,#3329,.T.);
#7475=EDGE_CURVE('',#6113,#6111,#3330,.T.);
#7476=EDGE_CURVE('',#6112,#6113,#3331,.T.);
#7477=EDGE_CURVE('',#6112,#6114,#3332,.T.);
#7478=EDGE_CURVE('',#6115,#6113,#3333,.T.);
#7479=EDGE_CURVE('',#6114,#6115,#3334,.T.);
#7480=EDGE_CURVE('',#6114,#6116,#3335,.T.);
#7481=EDGE_CURVE('',#6117,#6115,#3336,.T.);
#7482=EDGE_CURVE('',#6116,#6117,#3337,.T.);
#7483=EDGE_CURVE('',#6116,#6118,#3338,.T.);
#7484=EDGE_CURVE('',#6119,#6117,#3339,.T.);
#7485=EDGE_CURVE('',#6118,#6119,#3340,.T.);
#7486=EDGE_CURVE('',#6118,#6120,#3341,.T.);
#7487=EDGE_CURVE('',#6121,#6119,#3342,.T.);
#7488=EDGE_CURVE('',#6120,#6121,#3343,.T.);
#7489=EDGE_CURVE('',#6120,#6122,#3344,.T.);
#7490=EDGE_CURVE('',#6123,#6121,#3345,.T.);
#7491=EDGE_CURVE('',#6122,#6123,#3346,.T.);
#7492=EDGE_CURVE('',#6122,#6124,#3347,.T.);
#7493=EDGE_CURVE('',#6125,#6123,#3348,.T.);
#7494=EDGE_CURVE('',#6124,#6125,#3349,.T.);
#7495=EDGE_CURVE('',#6124,#6126,#3350,.T.);
#7496=EDGE_CURVE('',#6127,#6125,#3351,.T.);
#7497=EDGE_CURVE('',#6126,#6127,#3352,.T.);
#7498=EDGE_CURVE('',#6126,#6128,#3353,.T.);
#7499=EDGE_CURVE('',#6129,#6127,#3354,.T.);
#7500=EDGE_CURVE('',#6128,#6129,#3355,.T.);
#7501=EDGE_CURVE('',#6128,#6130,#3356,.T.);
#7502=EDGE_CURVE('',#6131,#6129,#3357,.T.);
#7503=EDGE_CURVE('',#6130,#6131,#3358,.T.);
#7504=EDGE_CURVE('',#6130,#6132,#3359,.T.);
#7505=EDGE_CURVE('',#6133,#6131,#3360,.T.);
#7506=EDGE_CURVE('',#6132,#6133,#3361,.T.);
#7507=EDGE_CURVE('',#6132,#6134,#3362,.T.);
#7508=EDGE_CURVE('',#6135,#6133,#3363,.T.);
#7509=EDGE_CURVE('',#6134,#6135,#3364,.T.);
#7510=EDGE_CURVE('',#6134,#6136,#3365,.T.);
#7511=EDGE_CURVE('',#6137,#6135,#3366,.T.);
#7512=EDGE_CURVE('',#6136,#6137,#3367,.T.);
#7513=EDGE_CURVE('',#6136,#6138,#3368,.T.);
#7514=EDGE_CURVE('',#6139,#6137,#3369,.T.);
#7515=EDGE_CURVE('',#6138,#6139,#3370,.T.);
#7516=EDGE_CURVE('',#6138,#6140,#3371,.T.);
#7517=EDGE_CURVE('',#6141,#6139,#3372,.T.);
#7518=EDGE_CURVE('',#6140,#6141,#3373,.T.);
#7519=EDGE_CURVE('',#6140,#6142,#3374,.T.);
#7520=EDGE_CURVE('',#6143,#6141,#3375,.T.);
#7521=EDGE_CURVE('',#6142,#6143,#3376,.T.);
#7522=EDGE_CURVE('',#6142,#6144,#3377,.T.);
#7523=EDGE_CURVE('',#6145,#6143,#3378,.T.);
#7524=EDGE_CURVE('',#6144,#6145,#3379,.T.);
#7525=EDGE_CURVE('',#6144,#6146,#3380,.T.);
#7526=EDGE_CURVE('',#6147,#6145,#3381,.T.);
#7527=EDGE_CURVE('',#6146,#6147,#3382,.T.);
#7528=EDGE_CURVE('',#6146,#6148,#3383,.T.);
#7529=EDGE_CURVE('',#6149,#6147,#3384,.T.);
#7530=EDGE_CURVE('',#6148,#6149,#3385,.T.);
#7531=EDGE_CURVE('',#6148,#6150,#3386,.T.);
#7532=EDGE_CURVE('',#6151,#6149,#3387,.T.);
#7533=EDGE_CURVE('',#6150,#6151,#3388,.T.);
#7534=EDGE_CURVE('',#6150,#6152,#3389,.T.);
#7535=EDGE_CURVE('',#6153,#6151,#3390,.T.);
#7536=EDGE_CURVE('',#6152,#6153,#3391,.T.);
#7537=EDGE_CURVE('',#6152,#6154,#3392,.T.);
#7538=EDGE_CURVE('',#6155,#6153,#3393,.T.);
#7539=EDGE_CURVE('',#6154,#6155,#3394,.T.);
#7540=EDGE_CURVE('',#6154,#6156,#3395,.T.);
#7541=EDGE_CURVE('',#6157,#6155,#3396,.T.);
#7542=EDGE_CURVE('',#6156,#6157,#3397,.T.);
#7543=EDGE_CURVE('',#6156,#6158,#3398,.T.);
#7544=EDGE_CURVE('',#6159,#6157,#3399,.T.);
#7545=EDGE_CURVE('',#6158,#6159,#3400,.T.);
#7546=EDGE_CURVE('',#6158,#6160,#3401,.T.);
#7547=EDGE_CURVE('',#6161,#6159,#3402,.T.);
#7548=EDGE_CURVE('',#6160,#6161,#3403,.T.);
#7549=EDGE_CURVE('',#6160,#6162,#3404,.T.);
#7550=EDGE_CURVE('',#6163,#6161,#3405,.T.);
#7551=EDGE_CURVE('',#6162,#6163,#3406,.T.);
#7552=EDGE_CURVE('',#6162,#6164,#3407,.T.);
#7553=EDGE_CURVE('',#6165,#6163,#3408,.T.);
#7554=EDGE_CURVE('',#6164,#6165,#3409,.T.);
#7555=EDGE_CURVE('',#6164,#6166,#3410,.T.);
#7556=EDGE_CURVE('',#6167,#6165,#3411,.T.);
#7557=EDGE_CURVE('',#6166,#6167,#3412,.T.);
#7558=EDGE_CURVE('',#6166,#6168,#3413,.T.);
#7559=EDGE_CURVE('',#6169,#6167,#3414,.T.);
#7560=EDGE_CURVE('',#6168,#6169,#3415,.T.);
#7561=EDGE_CURVE('',#6168,#6170,#3416,.T.);
#7562=EDGE_CURVE('',#6171,#6169,#3417,.T.);
#7563=EDGE_CURVE('',#6170,#6171,#3418,.T.);
#7564=EDGE_CURVE('',#6170,#6172,#3419,.T.);
#7565=EDGE_CURVE('',#6173,#6171,#3420,.T.);
#7566=EDGE_CURVE('',#6172,#6173,#3421,.T.);
#7567=EDGE_CURVE('',#6172,#6174,#3422,.T.);
#7568=EDGE_CURVE('',#6175,#6173,#3423,.T.);
#7569=EDGE_CURVE('',#6174,#6175,#3424,.T.);
#7570=EDGE_CURVE('',#6174,#6176,#3425,.T.);
#7571=EDGE_CURVE('',#6177,#6175,#3426,.T.);
#7572=EDGE_CURVE('',#6176,#6177,#3427,.T.);
#7573=EDGE_CURVE('',#6176,#6178,#3428,.T.);
#7574=EDGE_CURVE('',#6179,#6177,#3429,.T.);
#7575=EDGE_CURVE('',#6178,#6179,#3430,.T.);
#7576=EDGE_CURVE('',#6178,#6180,#3431,.T.);
#7577=EDGE_CURVE('',#6181,#6179,#3432,.T.);
#7578=EDGE_CURVE('',#6180,#6181,#3433,.T.);
#7579=EDGE_CURVE('',#6180,#6182,#3434,.T.);
#7580=EDGE_CURVE('',#6183,#6181,#3435,.T.);
#7581=EDGE_CURVE('',#6182,#6183,#3436,.T.);
#7582=EDGE_CURVE('',#6182,#6184,#3437,.T.);
#7583=EDGE_CURVE('',#6185,#6183,#3438,.T.);
#7584=EDGE_CURVE('',#6184,#6185,#3439,.T.);
#7585=EDGE_CURVE('',#6184,#6186,#3440,.T.);
#7586=EDGE_CURVE('',#6187,#6185,#3441,.T.);
#7587=EDGE_CURVE('',#6186,#6187,#3442,.T.);
#7588=EDGE_CURVE('',#6186,#6188,#3443,.T.);
#7589=EDGE_CURVE('',#6189,#6187,#3444,.T.);
#7590=EDGE_CURVE('',#6188,#6189,#3445,.T.);
#7591=EDGE_CURVE('',#6188,#6190,#3446,.T.);
#7592=EDGE_CURVE('',#6191,#6189,#3447,.T.);
#7593=EDGE_CURVE('',#6190,#6191,#3448,.T.);
#7594=EDGE_CURVE('',#6190,#6192,#3449,.T.);
#7595=EDGE_CURVE('',#6193,#6191,#3450,.T.);
#7596=EDGE_CURVE('',#6192,#6193,#3451,.T.);
#7597=EDGE_CURVE('',#6192,#6194,#3452,.T.);
#7598=EDGE_CURVE('',#6195,#6193,#3453,.T.);
#7599=EDGE_CURVE('',#6194,#6195,#3454,.T.);
#7600=EDGE_CURVE('',#6194,#6196,#3455,.T.);
#7601=EDGE_CURVE('',#6197,#6195,#3456,.T.);
#7602=EDGE_CURVE('',#6196,#6197,#3457,.T.);
#7603=EDGE_CURVE('',#6196,#6198,#3458,.T.);
#7604=EDGE_CURVE('',#6199,#6197,#3459,.T.);
#7605=EDGE_CURVE('',#6198,#6199,#3460,.T.);
#7606=EDGE_CURVE('',#6198,#6200,#3461,.T.);
#7607=EDGE_CURVE('',#6201,#6199,#3462,.T.);
#7608=EDGE_CURVE('',#6200,#6201,#3463,.T.);
#7609=EDGE_CURVE('',#6200,#6202,#3464,.T.);
#7610=EDGE_CURVE('',#6203,#6201,#3465,.T.);
#7611=EDGE_CURVE('',#6202,#6203,#3466,.T.);
#7612=EDGE_CURVE('',#6202,#6204,#3467,.T.);
#7613=EDGE_CURVE('',#6205,#6203,#3468,.T.);
#7614=EDGE_CURVE('',#6204,#6205,#3469,.T.);
#7615=EDGE_CURVE('',#6204,#6206,#3470,.T.);
#7616=EDGE_CURVE('',#6207,#6205,#3471,.T.);
#7617=EDGE_CURVE('',#6206,#6207,#3472,.T.);
#7618=EDGE_CURVE('',#6206,#6208,#3473,.T.);
#7619=EDGE_CURVE('',#6209,#6207,#3474,.T.);
#7620=EDGE_CURVE('',#6208,#6209,#3475,.T.);
#7621=EDGE_CURVE('',#6208,#6210,#3476,.T.);
#7622=EDGE_CURVE('',#6211,#6209,#3477,.T.);
#7623=EDGE_CURVE('',#6210,#6211,#3478,.T.);
#7624=EDGE_CURVE('',#6210,#6212,#3479,.T.);
#7625=EDGE_CURVE('',#6213,#6211,#3480,.T.);
#7626=EDGE_CURVE('',#6212,#6213,#3481,.T.);
#7627=EDGE_CURVE('',#6212,#6214,#3482,.T.);
#7628=EDGE_CURVE('',#6215,#6213,#3483,.T.);
#7629=EDGE_CURVE('',#6214,#6215,#3484,.T.);
#7630=EDGE_CURVE('',#6214,#6216,#3485,.T.);
#7631=EDGE_CURVE('',#6217,#6215,#3486,.T.);
#7632=EDGE_CURVE('',#6216,#6217,#3487,.T.);
#7633=EDGE_CURVE('',#6216,#6218,#3488,.T.);
#7634=EDGE_CURVE('',#6219,#6217,#3489,.T.);
#7635=EDGE_CURVE('',#6218,#6219,#3490,.T.);
#7636=EDGE_CURVE('',#6218,#6220,#3491,.T.);
#7637=EDGE_CURVE('',#6221,#6219,#3492,.T.);
#7638=EDGE_CURVE('',#6220,#6221,#3493,.T.);
#7639=EDGE_CURVE('',#6220,#6222,#3494,.T.);
#7640=EDGE_CURVE('',#6223,#6221,#3495,.T.);
#7641=EDGE_CURVE('',#6222,#6223,#3496,.T.);
#7642=EDGE_CURVE('',#6222,#6224,#3497,.T.);
#7643=EDGE_CURVE('',#6225,#6223,#3498,.T.);
#7644=EDGE_CURVE('',#6224,#6225,#3499,.T.);
#7645=EDGE_CURVE('',#6224,#6226,#3500,.T.);
#7646=EDGE_CURVE('',#6227,#6225,#3501,.T.);
#7647=EDGE_CURVE('',#6226,#6227,#3502,.T.);
#7648=EDGE_CURVE('',#6226,#6228,#3503,.T.);
#7649=EDGE_CURVE('',#6229,#6227,#3504,.T.);
#7650=EDGE_CURVE('',#6228,#6229,#3505,.T.);
#7651=EDGE_CURVE('',#6228,#6230,#3506,.T.);
#7652=EDGE_CURVE('',#6231,#6229,#3507,.T.);
#7653=EDGE_CURVE('',#6230,#6231,#3508,.T.);
#7654=EDGE_CURVE('',#6230,#6232,#3509,.T.);
#7655=EDGE_CURVE('',#6233,#6231,#3510,.T.);
#7656=EDGE_CURVE('',#6232,#6233,#3511,.T.);
#7657=EDGE_CURVE('',#6232,#6234,#3512,.T.);
#7658=EDGE_CURVE('',#6235,#6233,#3513,.T.);
#7659=EDGE_CURVE('',#6234,#6235,#3514,.T.);
#7660=EDGE_CURVE('',#6234,#6236,#3515,.T.);
#7661=EDGE_CURVE('',#6237,#6235,#3516,.T.);
#7662=EDGE_CURVE('',#6236,#6237,#3517,.T.);
#7663=EDGE_CURVE('',#6236,#6238,#3518,.T.);
#7664=EDGE_CURVE('',#6239,#6237,#3519,.T.);
#7665=EDGE_CURVE('',#6238,#6239,#3520,.T.);
#7666=EDGE_CURVE('',#6238,#6240,#3521,.T.);
#7667=EDGE_CURVE('',#6241,#6239,#3522,.T.);
#7668=EDGE_CURVE('',#6240,#6241,#3523,.T.);
#7669=EDGE_CURVE('',#6240,#6242,#3524,.T.);
#7670=EDGE_CURVE('',#6243,#6241,#3525,.T.);
#7671=EDGE_CURVE('',#6242,#6243,#3526,.T.);
#7672=EDGE_CURVE('',#6242,#6244,#3527,.T.);
#7673=EDGE_CURVE('',#6245,#6243,#3528,.T.);
#7674=EDGE_CURVE('',#6244,#6245,#3529,.T.);
#7675=EDGE_CURVE('',#6244,#6246,#3530,.T.);
#7676=EDGE_CURVE('',#6247,#6245,#3531,.T.);
#7677=EDGE_CURVE('',#6246,#6247,#3532,.T.);
#7678=EDGE_CURVE('',#6246,#6248,#3533,.T.);
#7679=EDGE_CURVE('',#6249,#6247,#3534,.T.);
#7680=EDGE_CURVE('',#6248,#6249,#3535,.T.);
#7681=EDGE_CURVE('',#6248,#6250,#3536,.T.);
#7682=EDGE_CURVE('',#6251,#6249,#3537,.T.);
#7683=EDGE_CURVE('',#6250,#6251,#3538,.T.);
#7684=EDGE_CURVE('',#6250,#6252,#3539,.T.);
#7685=EDGE_CURVE('',#6253,#6251,#3540,.T.);
#7686=EDGE_CURVE('',#6252,#6253,#3541,.T.);
#7687=EDGE_CURVE('',#6252,#6254,#3542,.T.);
#7688=EDGE_CURVE('',#6255,#6253,#3543,.T.);
#7689=EDGE_CURVE('',#6254,#6255,#3544,.T.);
#7690=EDGE_CURVE('',#6254,#6256,#3545,.T.);
#7691=EDGE_CURVE('',#6257,#6255,#3546,.T.);
#7692=EDGE_CURVE('',#6256,#6257,#3547,.T.);
#7693=EDGE_CURVE('',#6256,#6258,#3548,.T.);
#7694=EDGE_CURVE('',#6259,#6257,#3549,.T.);
#7695=EDGE_CURVE('',#6258,#6259,#3550,.T.);
#7696=EDGE_CURVE('',#6258,#6260,#3551,.T.);
#7697=EDGE_CURVE('',#6261,#6259,#3552,.T.);
#7698=EDGE_CURVE('',#6260,#6261,#3553,.T.);
#7699=EDGE_CURVE('',#6260,#6262,#3554,.T.);
#7700=EDGE_CURVE('',#6263,#6261,#3555,.T.);
#7701=EDGE_CURVE('',#6262,#6263,#3556,.T.);
#7702=EDGE_CURVE('',#6262,#6264,#3557,.T.);
#7703=EDGE_CURVE('',#6265,#6263,#3558,.T.);
#7704=EDGE_CURVE('',#6264,#6265,#3559,.T.);
#7705=EDGE_CURVE('',#6264,#6266,#3560,.T.);
#7706=EDGE_CURVE('',#6267,#6265,#3561,.T.);
#7707=EDGE_CURVE('',#6266,#6267,#3562,.T.);
#7708=EDGE_CURVE('',#6266,#6268,#3563,.T.);
#7709=EDGE_CURVE('',#6269,#6267,#3564,.T.);
#7710=EDGE_CURVE('',#6268,#6269,#3565,.T.);
#7711=EDGE_CURVE('',#6268,#6270,#3566,.T.);
#7712=EDGE_CURVE('',#6271,#6269,#3567,.T.);
#7713=EDGE_CURVE('',#6270,#6271,#3568,.T.);
#7714=EDGE_CURVE('',#6270,#6272,#3569,.T.);
#7715=EDGE_CURVE('',#6273,#6271,#3570,.T.);
#7716=EDGE_CURVE('',#6272,#6273,#3571,.T.);
#7717=EDGE_CURVE('',#6272,#6274,#3572,.T.);
#7718=EDGE_CURVE('',#6275,#6273,#3573,.T.);
#7719=EDGE_CURVE('',#6274,#6275,#3574,.T.);
#7720=EDGE_CURVE('',#6274,#6276,#3575,.T.);
#7721=EDGE_CURVE('',#6277,#6275,#3576,.T.);
#7722=EDGE_CURVE('',#6276,#6277,#3577,.T.);
#7723=EDGE_CURVE('',#6276,#6278,#3578,.T.);
#7724=EDGE_CURVE('',#6279,#6277,#3579,.T.);
#7725=EDGE_CURVE('',#6278,#6279,#3580,.T.);
#7726=EDGE_CURVE('',#6278,#6280,#3581,.T.);
#7727=EDGE_CURVE('',#6281,#6279,#3582,.T.);
#7728=EDGE_CURVE('',#6280,#6281,#3583,.T.);
#7729=EDGE_CURVE('',#6280,#6282,#3584,.T.);
#7730=EDGE_CURVE('',#6283,#6281,#3585,.T.);
#7731=EDGE_CURVE('',#6282,#6283,#3586,.T.);
#7732=EDGE_CURVE('',#6282,#6284,#3587,.T.);
#7733=EDGE_CURVE('',#6285,#6283,#3588,.T.);
#7734=EDGE_CURVE('',#6284,#6285,#3589,.T.);
#7735=EDGE_CURVE('',#6284,#6286,#3590,.T.);
#7736=EDGE_CURVE('',#6287,#6285,#3591,.T.);
#7737=EDGE_CURVE('',#6286,#6287,#3592,.T.);
#7738=EDGE_CURVE('',#6286,#6288,#3593,.T.);
#7739=EDGE_CURVE('',#6289,#6287,#3594,.T.);
#7740=EDGE_CURVE('',#6288,#6289,#3595,.T.);
#7741=EDGE_CURVE('',#6288,#6290,#3596,.T.);
#7742=EDGE_CURVE('',#6291,#6289,#3597,.T.);
#7743=EDGE_CURVE('',#6290,#6291,#3598,.T.);
#7744=EDGE_CURVE('',#6290,#6292,#3599,.T.);
#7745=EDGE_CURVE('',#6293,#6291,#3600,.T.);
#7746=EDGE_CURVE('',#6292,#6293,#3601,.T.);
#7747=EDGE_CURVE('',#6292,#6294,#3602,.T.);
#7748=EDGE_CURVE('',#6295,#6293,#3603,.T.);
#7749=EDGE_CURVE('',#6294,#6295,#3604,.T.);
#7750=EDGE_CURVE('',#6294,#6296,#3605,.T.);
#7751=EDGE_CURVE('',#6297,#6295,#3606,.T.);
#7752=EDGE_CURVE('',#6296,#6297,#3607,.T.);
#7753=EDGE_CURVE('',#6296,#6298,#3608,.T.);
#7754=EDGE_CURVE('',#6299,#6297,#3609,.T.);
#7755=EDGE_CURVE('',#6298,#6299,#3610,.T.);
#7756=EDGE_CURVE('',#6298,#6300,#3611,.T.);
#7757=EDGE_CURVE('',#6301,#6299,#3612,.T.);
#7758=EDGE_CURVE('',#6300,#6301,#3613,.T.);
#7759=EDGE_CURVE('',#6300,#6302,#3614,.T.);
#7760=EDGE_CURVE('',#6303,#6301,#3615,.T.);
#7761=EDGE_CURVE('',#6302,#6303,#3616,.T.);
#7762=EDGE_CURVE('',#6302,#6304,#3617,.T.);
#7763=EDGE_CURVE('',#6305,#6303,#3618,.T.);
#7764=EDGE_CURVE('',#6304,#6305,#3619,.T.);
#7765=EDGE_CURVE('',#6304,#6306,#3620,.T.);
#7766=EDGE_CURVE('',#6307,#6305,#3621,.T.);
#7767=EDGE_CURVE('',#6306,#6307,#3622,.T.);
#7768=EDGE_CURVE('',#6306,#6308,#3623,.T.);
#7769=EDGE_CURVE('',#6309,#6307,#3624,.T.);
#7770=EDGE_CURVE('',#6308,#6309,#3625,.T.);
#7771=EDGE_CURVE('',#6308,#6310,#3626,.T.);
#7772=EDGE_CURVE('',#6311,#6309,#3627,.T.);
#7773=EDGE_CURVE('',#6310,#6311,#3628,.T.);
#7774=EDGE_CURVE('',#6310,#6312,#3629,.T.);
#7775=EDGE_CURVE('',#6313,#6311,#3630,.T.);
#7776=EDGE_CURVE('',#6312,#6313,#3631,.T.);
#7777=EDGE_CURVE('',#6312,#6314,#3632,.T.);
#7778=EDGE_CURVE('',#6315,#6313,#3633,.T.);
#7779=EDGE_CURVE('',#6314,#6315,#3634,.T.);
#7780=EDGE_CURVE('',#6314,#6316,#3635,.T.);
#7781=EDGE_CURVE('',#6317,#6315,#3636,.T.);
#7782=EDGE_CURVE('',#6316,#6317,#3637,.T.);
#7783=EDGE_CURVE('',#6316,#6318,#3638,.T.);
#7784=EDGE_CURVE('',#6319,#6317,#3639,.T.);
#7785=EDGE_CURVE('',#6318,#6319,#3640,.T.);
#7786=EDGE_CURVE('',#6318,#6320,#3641,.T.);
#7787=EDGE_CURVE('',#6321,#6319,#3642,.T.);
#7788=EDGE_CURVE('',#6320,#6321,#3643,.T.);
#7789=EDGE_CURVE('',#6320,#6322,#3644,.T.);
#7790=EDGE_CURVE('',#6323,#6321,#3645,.T.);
#7791=EDGE_CURVE('',#6322,#6323,#3646,.T.);
#7792=EDGE_CURVE('',#6322,#6324,#3647,.T.);
#7793=EDGE_CURVE('',#6325,#6323,#3648,.T.);
#7794=EDGE_CURVE('',#6324,#6325,#3649,.T.);
#7795=EDGE_CURVE('',#6324,#6326,#3650,.T.);
#7796=EDGE_CURVE('',#6327,#6325,#3651,.T.);
#7797=EDGE_CURVE('',#6326,#6327,#3652,.T.);
#7798=EDGE_CURVE('',#6326,#6328,#3653,.T.);
#7799=EDGE_CURVE('',#6329,#6327,#3654,.T.);
#7800=EDGE_CURVE('',#6328,#6329,#3655,.T.);
#7801=EDGE_CURVE('',#6328,#6330,#3656,.T.);
#7802=EDGE_CURVE('',#6331,#6329,#3657,.T.);
#7803=EDGE_CURVE('',#6330,#6331,#3658,.T.);
#7804=EDGE_CURVE('',#6330,#6332,#3659,.T.);
#7805=EDGE_CURVE('',#6333,#6331,#3660,.T.);
#7806=EDGE_CURVE('',#6332,#6333,#3661,.T.);
#7807=EDGE_CURVE('',#6332,#6334,#3662,.T.);
#7808=EDGE_CURVE('',#6335,#6333,#3663,.T.);
#7809=EDGE_CURVE('',#6334,#6335,#3664,.T.);
#7810=EDGE_CURVE('',#6334,#6336,#3665,.T.);
#7811=EDGE_CURVE('',#6337,#6335,#3666,.T.);
#7812=EDGE_CURVE('',#6336,#6337,#3667,.T.);
#7813=EDGE_CURVE('',#6336,#6338,#3668,.T.);
#7814=EDGE_CURVE('',#6339,#6337,#3669,.T.);
#7815=EDGE_CURVE('',#6338,#6339,#3670,.T.);
#7816=EDGE_CURVE('',#6338,#6340,#3671,.T.);
#7817=EDGE_CURVE('',#6341,#6339,#3672,.T.);
#7818=EDGE_CURVE('',#6340,#6341,#3673,.T.);
#7819=EDGE_CURVE('',#6340,#6342,#3674,.T.);
#7820=EDGE_CURVE('',#6343,#6341,#3675,.T.);
#7821=EDGE_CURVE('',#6342,#6343,#3676,.T.);
#7822=EDGE_CURVE('',#6342,#6344,#3677,.T.);
#7823=EDGE_CURVE('',#6345,#6343,#3678,.T.);
#7824=EDGE_CURVE('',#6344,#6345,#3679,.T.);
#7825=EDGE_CURVE('',#6344,#6346,#3680,.T.);
#7826=EDGE_CURVE('',#6347,#6345,#3681,.T.);
#7827=EDGE_CURVE('',#6346,#6347,#3682,.T.);
#7828=EDGE_CURVE('',#6346,#6348,#3683,.T.);
#7829=EDGE_CURVE('',#6349,#6347,#3684,.T.);
#7830=EDGE_CURVE('',#6348,#6349,#3685,.T.);
#7831=EDGE_CURVE('',#6348,#6350,#3686,.T.);
#7832=EDGE_CURVE('',#6351,#6349,#3687,.T.);
#7833=EDGE_CURVE('',#6350,#6351,#3688,.T.);
#7834=EDGE_CURVE('',#6350,#6352,#3689,.T.);
#7835=EDGE_CURVE('',#6353,#6351,#3690,.T.);
#7836=EDGE_CURVE('',#6352,#6353,#3691,.T.);
#7837=EDGE_CURVE('',#6352,#6354,#3692,.T.);
#7838=EDGE_CURVE('',#6355,#6353,#3693,.T.);
#7839=EDGE_CURVE('',#6354,#6355,#3694,.T.);
#7840=EDGE_CURVE('',#6354,#6356,#3695,.T.);
#7841=EDGE_CURVE('',#6357,#6355,#3696,.T.);
#7842=EDGE_CURVE('',#6356,#6357,#3697,.T.);
#7843=EDGE_CURVE('',#6356,#6358,#3698,.T.);
#7844=EDGE_CURVE('',#6359,#6357,#3699,.T.);
#7845=EDGE_CURVE('',#6358,#6359,#3700,.T.);
#7846=EDGE_CURVE('',#6358,#6360,#3701,.T.);
#7847=EDGE_CURVE('',#6361,#6359,#3702,.T.);
#7848=EDGE_CURVE('',#6360,#6361,#3703,.T.);
#7849=EDGE_CURVE('',#6360,#6362,#3704,.T.);
#7850=EDGE_CURVE('',#6363,#6361,#3705,.T.);
#7851=EDGE_CURVE('',#6362,#6363,#3706,.T.);
#7852=EDGE_CURVE('',#6362,#6364,#3707,.T.);
#7853=EDGE_CURVE('',#6365,#6363,#3708,.T.);
#7854=EDGE_CURVE('',#6364,#6365,#3709,.T.);
#7855=EDGE_CURVE('',#6364,#6366,#3710,.T.);
#7856=EDGE_CURVE('',#6367,#6365,#3711,.T.);
#7857=EDGE_CURVE('',#6366,#6367,#3712,.T.);
#7858=EDGE_CURVE('',#6366,#6368,#3713,.T.);
#7859=EDGE_CURVE('',#6369,#6367,#3714,.T.);
#7860=EDGE_CURVE('',#6368,#6369,#3715,.T.);
#7861=EDGE_CURVE('',#6368,#6370,#3716,.T.);
#7862=EDGE_CURVE('',#6371,#6369,#3717,.T.);
#7863=EDGE_CURVE('',#6370,#6371,#3718,.T.);
#7864=EDGE_CURVE('',#6370,#6372,#3719,.T.);
#7865=EDGE_CURVE('',#6373,#6371,#3720,.T.);
#7866=EDGE_CURVE('',#6372,#6373,#3721,.T.);
#7867=EDGE_CURVE('',#6372,#6374,#3722,.T.);
#7868=EDGE_CURVE('',#6375,#6373,#3723,.T.);
#7869=EDGE_CURVE('',#6374,#6375,#3724,.T.);
#7870=EDGE_CURVE('',#6374,#6376,#3725,.T.);
#7871=EDGE_CURVE('',#6377,#6375,#3726,.T.);
#7872=EDGE_CURVE('',#6376,#6377,#3727,.T.);
#7873=EDGE_CURVE('',#6376,#6378,#3728,.T.);
#7874=EDGE_CURVE('',#6379,#6377,#3729,.T.);
#7875=EDGE_CURVE('',#6378,#6379,#3730,.T.);
#7876=EDGE_CURVE('',#6378,#6380,#3731,.T.);
#7877=EDGE_CURVE('',#6381,#6379,#3732,.T.);
#7878=EDGE_CURVE('',#6380,#6381,#3733,.T.);
#7879=EDGE_CURVE('',#6380,#6382,#3734,.T.);
#7880=EDGE_CURVE('',#6383,#6381,#3735,.T.);
#7881=EDGE_CURVE('',#6382,#6383,#3736,.T.);
#7882=EDGE_CURVE('',#6382,#6059,#3737,.T.);
#7883=EDGE_CURVE('',#6060,#6383,#3738,.T.);
#7884=EDGE_CURVE('',#6384,#6384,#5475,.T.);
#7885=EDGE_CURVE('',#6384,#6061,#3739,.T.);
#7886=EDGE_CURVE('',#6058,#6385,#3740,.T.);
#7887=EDGE_CURVE('',#6385,#6385,#5476,.T.);
#9705=ORIENTED_EDGE('',*,*,#7381,.F.);
#9706=ORIENTED_EDGE('',*,*,#7382,.T.);
#9707=ORIENTED_EDGE('',*,*,#7383,.T.);
#9708=ORIENTED_EDGE('',*,*,#7382,.F.);
#9709=ORIENTED_EDGE('',*,*,#7383,.F.);
#9710=ORIENTED_EDGE('',*,*,#7384,.F.);
#9711=ORIENTED_EDGE('',*,*,#7385,.F.);
#9712=ORIENTED_EDGE('',*,*,#7386,.F.);
#9713=ORIENTED_EDGE('',*,*,#7387,.T.);
#9714=ORIENTED_EDGE('',*,*,#7388,.F.);
#9715=ORIENTED_EDGE('',*,*,#7389,.T.);
#9716=ORIENTED_EDGE('',*,*,#7390,.F.);
#9717=ORIENTED_EDGE('',*,*,#7391,.F.);
#9718=ORIENTED_EDGE('',*,*,#7392,.F.);
#9719=ORIENTED_EDGE('',*,*,#7387,.F.);
#9720=ORIENTED_EDGE('',*,*,#7393,.F.);
#9721=ORIENTED_EDGE('',*,*,#7394,.T.);
#9722=ORIENTED_EDGE('',*,*,#7395,.F.);
#9723=ORIENTED_EDGE('',*,*,#7389,.F.);
#9724=ORIENTED_EDGE('',*,*,#7396,.F.);
#9725=ORIENTED_EDGE('',*,*,#7397,.F.);
#9726=ORIENTED_EDGE('',*,*,#7391,.T.);
#9727=ORIENTED_EDGE('',*,*,#7398,.F.);
#9728=ORIENTED_EDGE('',*,*,#7399,.F.);
#9729=ORIENTED_EDGE('',*,*,#7400,.F.);
#9730=ORIENTED_EDGE('',*,*,#7385,.T.);
#9731=ORIENTED_EDGE('',*,*,#7401,.F.);
#9732=ORIENTED_EDGE('',*,*,#7402,.F.);
#9733=ORIENTED_EDGE('',*,*,#7399,.T.);
#9734=ORIENTED_EDGE('',*,*,#7403,.F.);
#9735=ORIENTED_EDGE('',*,*,#7404,.F.);
#9736=ORIENTED_EDGE('',*,*,#7405,.F.);
#9737=ORIENTED_EDGE('',*,*,#7404,.T.);
#9738=ORIENTED_EDGE('',*,*,#7406,.F.);
#9739=ORIENTED_EDGE('',*,*,#7407,.F.);
#9740=ORIENTED_EDGE('',*,*,#7408,.F.);
#9741=ORIENTED_EDGE('',*,*,#7407,.T.);
#9742=ORIENTED_EDGE('',*,*,#7409,.F.);
#9743=ORIENTED_EDGE('',*,*,#7410,.F.);
#9744=ORIENTED_EDGE('',*,*,#7411,.F.);
#9745=ORIENTED_EDGE('',*,*,#7410,.T.);
#9746=ORIENTED_EDGE('',*,*,#7412,.F.);
#9747=ORIENTED_EDGE('',*,*,#7413,.F.);
#9748=ORIENTED_EDGE('',*,*,#7414,.F.);
#9749=ORIENTED_EDGE('',*,*,#7413,.T.);
#9750=ORIENTED_EDGE('',*,*,#7415,.F.);
#9751=ORIENTED_EDGE('',*,*,#7416,.F.);
#9752=ORIENTED_EDGE('',*,*,#7417,.F.);
#9753=ORIENTED_EDGE('',*,*,#7416,.T.);
#9754=ORIENTED_EDGE('',*,*,#7418,.F.);
#9755=ORIENTED_EDGE('',*,*,#7419,.F.);
#9756=ORIENTED_EDGE('',*,*,#7420,.F.);
#9757=ORIENTED_EDGE('',*,*,#7419,.T.);
#9758=ORIENTED_EDGE('',*,*,#7421,.F.);
#9759=ORIENTED_EDGE('',*,*,#7422,.F.);
#9760=ORIENTED_EDGE('',*,*,#7423,.F.);
#9761=ORIENTED_EDGE('',*,*,#7422,.T.);
#9762=ORIENTED_EDGE('',*,*,#7424,.F.);
#9763=ORIENTED_EDGE('',*,*,#7425,.F.);
#9764=ORIENTED_EDGE('',*,*,#7426,.F.);
#9765=ORIENTED_EDGE('',*,*,#7425,.T.);
#9766=ORIENTED_EDGE('',*,*,#7427,.F.);
#9767=ORIENTED_EDGE('',*,*,#7428,.F.);
#9768=ORIENTED_EDGE('',*,*,#7429,.F.);
#9769=ORIENTED_EDGE('',*,*,#7428,.T.);
#9770=ORIENTED_EDGE('',*,*,#7430,.F.);
#9771=ORIENTED_EDGE('',*,*,#7431,.F.);
#9772=ORIENTED_EDGE('',*,*,#7432,.F.);
#9773=ORIENTED_EDGE('',*,*,#7431,.T.);
#9774=ORIENTED_EDGE('',*,*,#7433,.F.);
#9775=ORIENTED_EDGE('',*,*,#7434,.F.);
#9776=ORIENTED_EDGE('',*,*,#7435,.F.);
#9777=ORIENTED_EDGE('',*,*,#7434,.T.);
#9778=ORIENTED_EDGE('',*,*,#7436,.F.);
#9779=ORIENTED_EDGE('',*,*,#7437,.F.);
#9780=ORIENTED_EDGE('',*,*,#7438,.F.);
#9781=ORIENTED_EDGE('',*,*,#7437,.T.);
#9782=ORIENTED_EDGE('',*,*,#7439,.F.);
#9783=ORIENTED_EDGE('',*,*,#7440,.F.);
#9784=ORIENTED_EDGE('',*,*,#7441,.F.);
#9785=ORIENTED_EDGE('',*,*,#7440,.T.);
#9786=ORIENTED_EDGE('',*,*,#7442,.F.);
#9787=ORIENTED_EDGE('',*,*,#7443,.F.);
#9788=ORIENTED_EDGE('',*,*,#7444,.F.);
#9789=ORIENTED_EDGE('',*,*,#7443,.T.);
#9790=ORIENTED_EDGE('',*,*,#7445,.F.);
#9791=ORIENTED_EDGE('',*,*,#7446,.F.);
#9792=ORIENTED_EDGE('',*,*,#7447,.F.);
#9793=ORIENTED_EDGE('',*,*,#7446,.T.);
#9794=ORIENTED_EDGE('',*,*,#7448,.F.);
#9795=ORIENTED_EDGE('',*,*,#7449,.F.);
#9796=ORIENTED_EDGE('',*,*,#7450,.F.);
#9797=ORIENTED_EDGE('',*,*,#7449,.T.);
#9798=ORIENTED_EDGE('',*,*,#7451,.F.);
#9799=ORIENTED_EDGE('',*,*,#7452,.F.);
#9800=ORIENTED_EDGE('',*,*,#7453,.F.);
#9801=ORIENTED_EDGE('',*,*,#7452,.T.);
#9802=ORIENTED_EDGE('',*,*,#7454,.F.);
#9803=ORIENTED_EDGE('',*,*,#7455,.F.);
#9804=ORIENTED_EDGE('',*,*,#7456,.F.);
#9805=ORIENTED_EDGE('',*,*,#7455,.T.);
#9806=ORIENTED_EDGE('',*,*,#7457,.F.);
#9807=ORIENTED_EDGE('',*,*,#7458,.F.);
#9808=ORIENTED_EDGE('',*,*,#7459,.F.);
#9809=ORIENTED_EDGE('',*,*,#7458,.T.);
#9810=ORIENTED_EDGE('',*,*,#7460,.F.);
#9811=ORIENTED_EDGE('',*,*,#7461,.F.);
#9812=ORIENTED_EDGE('',*,*,#7462,.F.);
#9813=ORIENTED_EDGE('',*,*,#7461,.T.);
#9814=ORIENTED_EDGE('',*,*,#7463,.F.);
#9815=ORIENTED_EDGE('',*,*,#7464,.F.);
#9816=ORIENTED_EDGE('',*,*,#7465,.F.);
#9817=ORIENTED_EDGE('',*,*,#7464,.T.);
#9818=ORIENTED_EDGE('',*,*,#7466,.F.);
#9819=ORIENTED_EDGE('',*,*,#7467,.F.);
#9820=ORIENTED_EDGE('',*,*,#7468,.F.);
#9821=ORIENTED_EDGE('',*,*,#7467,.T.);
#9822=ORIENTED_EDGE('',*,*,#7469,.F.);
#9823=ORIENTED_EDGE('',*,*,#7470,.F.);
#9824=ORIENTED_EDGE('',*,*,#7471,.F.);
#9825=ORIENTED_EDGE('',*,*,#7470,.T.);
#9826=ORIENTED_EDGE('',*,*,#7472,.F.);
#9827=ORIENTED_EDGE('',*,*,#7473,.F.);
#9828=ORIENTED_EDGE('',*,*,#7474,.F.);
#9829=ORIENTED_EDGE('',*,*,#7473,.T.);
#9830=ORIENTED_EDGE('',*,*,#7475,.F.);
#9831=ORIENTED_EDGE('',*,*,#7476,.F.);
#9832=ORIENTED_EDGE('',*,*,#7477,.F.);
#9833=ORIENTED_EDGE('',*,*,#7476,.T.);
#9834=ORIENTED_EDGE('',*,*,#7478,.F.);
#9835=ORIENTED_EDGE('',*,*,#7479,.F.);
#9836=ORIENTED_EDGE('',*,*,#7480,.F.);
#9837=ORIENTED_EDGE('',*,*,#7479,.T.);
#9838=ORIENTED_EDGE('',*,*,#7481,.F.);
#9839=ORIENTED_EDGE('',*,*,#7482,.F.);
#9840=ORIENTED_EDGE('',*,*,#7483,.F.);
#9841=ORIENTED_EDGE('',*,*,#7482,.T.);
#9842=ORIENTED_EDGE('',*,*,#7484,.F.);
#9843=ORIENTED_EDGE('',*,*,#7485,.F.);
#9844=ORIENTED_EDGE('',*,*,#7486,.F.);
#9845=ORIENTED_EDGE('',*,*,#7485,.T.);
#9846=ORIENTED_EDGE('',*,*,#7487,.F.);
#9847=ORIENTED_EDGE('',*,*,#7488,.F.);
#9848=ORIENTED_EDGE('',*,*,#7489,.F.);
#9849=ORIENTED_EDGE('',*,*,#7488,.T.);
#9850=ORIENTED_EDGE('',*,*,#7490,.F.);
#9851=ORIENTED_EDGE('',*,*,#7491,.F.);
#9852=ORIENTED_EDGE('',*,*,#7492,.F.);
#9853=ORIENTED_EDGE('',*,*,#7491,.T.);
#9854=ORIENTED_EDGE('',*,*,#7493,.F.);
#9855=ORIENTED_EDGE('',*,*,#7494,.F.);
#9856=ORIENTED_EDGE('',*,*,#7495,.F.);
#9857=ORIENTED_EDGE('',*,*,#7494,.T.);
#9858=ORIENTED_EDGE('',*,*,#7496,.F.);
#9859=ORIENTED_EDGE('',*,*,#7497,.F.);
#9860=ORIENTED_EDGE('',*,*,#7498,.F.);
#9861=ORIENTED_EDGE('',*,*,#7497,.T.);
#9862=ORIENTED_EDGE('',*,*,#7499,.F.);
#9863=ORIENTED_EDGE('',*,*,#7500,.F.);
#9864=ORIENTED_EDGE('',*,*,#7501,.F.);
#9865=ORIENTED_EDGE('',*,*,#7500,.T.);
#9866=ORIENTED_EDGE('',*,*,#7502,.F.);
#9867=ORIENTED_EDGE('',*,*,#7503,.F.);
#9868=ORIENTED_EDGE('',*,*,#7504,.F.);
#9869=ORIENTED_EDGE('',*,*,#7503,.T.);
#9870=ORIENTED_EDGE('',*,*,#7505,.F.);
#9871=ORIENTED_EDGE('',*,*,#7506,.F.);
#9872=ORIENTED_EDGE('',*,*,#7507,.F.);
#9873=ORIENTED_EDGE('',*,*,#7506,.T.);
#9874=ORIENTED_EDGE('',*,*,#7508,.F.);
#9875=ORIENTED_EDGE('',*,*,#7509,.F.);
#9876=ORIENTED_EDGE('',*,*,#7510,.F.);
#9877=ORIENTED_EDGE('',*,*,#7509,.T.);
#9878=ORIENTED_EDGE('',*,*,#7511,.F.);
#9879=ORIENTED_EDGE('',*,*,#7512,.F.);
#9880=ORIENTED_EDGE('',*,*,#7513,.F.);
#9881=ORIENTED_EDGE('',*,*,#7512,.T.);
#9882=ORIENTED_EDGE('',*,*,#7514,.F.);
#9883=ORIENTED_EDGE('',*,*,#7515,.F.);
#9884=ORIENTED_EDGE('',*,*,#7516,.F.);
#9885=ORIENTED_EDGE('',*,*,#7515,.T.);
#9886=ORIENTED_EDGE('',*,*,#7517,.F.);
#9887=ORIENTED_EDGE('',*,*,#7518,.F.);
#9888=ORIENTED_EDGE('',*,*,#7519,.F.);
#9889=ORIENTED_EDGE('',*,*,#7518,.T.);
#9890=ORIENTED_EDGE('',*,*,#7520,.F.);
#9891=ORIENTED_EDGE('',*,*,#7521,.F.);
#9892=ORIENTED_EDGE('',*,*,#7522,.F.);
#9893=ORIENTED_EDGE('',*,*,#7521,.T.);
#9894=ORIENTED_EDGE('',*,*,#7523,.F.);
#9895=ORIENTED_EDGE('',*,*,#7524,.F.);
#9896=ORIENTED_EDGE('',*,*,#7525,.F.);
#9897=ORIENTED_EDGE('',*,*,#7524,.T.);
#9898=ORIENTED_EDGE('',*,*,#7526,.F.);
#9899=ORIENTED_EDGE('',*,*,#7527,.F.);
#9900=ORIENTED_EDGE('',*,*,#7528,.F.);
#9901=ORIENTED_EDGE('',*,*,#7527,.T.);
#9902=ORIENTED_EDGE('',*,*,#7529,.F.);
#9903=ORIENTED_EDGE('',*,*,#7530,.F.);
#9904=ORIENTED_EDGE('',*,*,#7531,.F.);
#9905=ORIENTED_EDGE('',*,*,#7530,.T.);
#9906=ORIENTED_EDGE('',*,*,#7532,.F.);
#9907=ORIENTED_EDGE('',*,*,#7533,.F.);
#9908=ORIENTED_EDGE('',*,*,#7534,.F.);
#9909=ORIENTED_EDGE('',*,*,#7533,.T.);
#9910=ORIENTED_EDGE('',*,*,#7535,.F.);
#9911=ORIENTED_EDGE('',*,*,#7536,.F.);
#9912=ORIENTED_EDGE('',*,*,#7537,.F.);
#9913=ORIENTED_EDGE('',*,*,#7536,.T.);
#9914=ORIENTED_EDGE('',*,*,#7538,.F.);
#9915=ORIENTED_EDGE('',*,*,#7539,.F.);
#9916=ORIENTED_EDGE('',*,*,#7540,.F.);
#9917=ORIENTED_EDGE('',*,*,#7539,.T.);
#9918=ORIENTED_EDGE('',*,*,#7541,.F.);
#9919=ORIENTED_EDGE('',*,*,#7542,.F.);
#9920=ORIENTED_EDGE('',*,*,#7543,.F.);
#9921=ORIENTED_EDGE('',*,*,#7542,.T.);
#9922=ORIENTED_EDGE('',*,*,#7544,.F.);
#9923=ORIENTED_EDGE('',*,*,#7545,.F.);
#9924=ORIENTED_EDGE('',*,*,#7546,.F.);
#9925=ORIENTED_EDGE('',*,*,#7545,.T.);
#9926=ORIENTED_EDGE('',*,*,#7547,.F.);
#9927=ORIENTED_EDGE('',*,*,#7548,.F.);
#9928=ORIENTED_EDGE('',*,*,#7549,.F.);
#9929=ORIENTED_EDGE('',*,*,#7548,.T.);
#9930=ORIENTED_EDGE('',*,*,#7550,.F.);
#9931=ORIENTED_EDGE('',*,*,#7551,.F.);
#9932=ORIENTED_EDGE('',*,*,#7552,.F.);
#9933=ORIENTED_EDGE('',*,*,#7551,.T.);
#9934=ORIENTED_EDGE('',*,*,#7553,.F.);
#9935=ORIENTED_EDGE('',*,*,#7554,.F.);
#9936=ORIENTED_EDGE('',*,*,#7555,.F.);
#9937=ORIENTED_EDGE('',*,*,#7554,.T.);
#9938=ORIENTED_EDGE('',*,*,#7556,.F.);
#9939=ORIENTED_EDGE('',*,*,#7557,.F.);
#9940=ORIENTED_EDGE('',*,*,#7558,.F.);
#9941=ORIENTED_EDGE('',*,*,#7557,.T.);
#9942=ORIENTED_EDGE('',*,*,#7559,.F.);
#9943=ORIENTED_EDGE('',*,*,#7560,.F.);
#9944=ORIENTED_EDGE('',*,*,#7561,.F.);
#9945=ORIENTED_EDGE('',*,*,#7560,.T.);
#9946=ORIENTED_EDGE('',*,*,#7562,.F.);
#9947=ORIENTED_EDGE('',*,*,#7563,.F.);
#9948=ORIENTED_EDGE('',*,*,#7564,.F.);
#9949=ORIENTED_EDGE('',*,*,#7563,.T.);
#9950=ORIENTED_EDGE('',*,*,#7565,.F.);
#9951=ORIENTED_EDGE('',*,*,#7566,.F.);
#9952=ORIENTED_EDGE('',*,*,#7567,.F.);
#9953=ORIENTED_EDGE('',*,*,#7566,.T.);
#9954=ORIENTED_EDGE('',*,*,#7568,.F.);
#9955=ORIENTED_EDGE('',*,*,#7569,.F.);
#9956=ORIENTED_EDGE('',*,*,#7570,.F.);
#9957=ORIENTED_EDGE('',*,*,#7569,.T.);
#9958=ORIENTED_EDGE('',*,*,#7571,.F.);
#9959=ORIENTED_EDGE('',*,*,#7572,.F.);
#9960=ORIENTED_EDGE('',*,*,#7573,.F.);
#9961=ORIENTED_EDGE('',*,*,#7572,.T.);
#9962=ORIENTED_EDGE('',*,*,#7574,.F.);
#9963=ORIENTED_EDGE('',*,*,#7575,.F.);
#9964=ORIENTED_EDGE('',*,*,#7576,.F.);
#9965=ORIENTED_EDGE('',*,*,#7575,.T.);
#9966=ORIENTED_EDGE('',*,*,#7577,.F.);
#9967=ORIENTED_EDGE('',*,*,#7578,.F.);
#9968=ORIENTED_EDGE('',*,*,#7579,.F.);
#9969=ORIENTED_EDGE('',*,*,#7578,.T.);
#9970=ORIENTED_EDGE('',*,*,#7580,.F.);
#9971=ORIENTED_EDGE('',*,*,#7581,.F.);
#9972=ORIENTED_EDGE('',*,*,#7582,.F.);
#9973=ORIENTED_EDGE('',*,*,#7581,.T.);
#9974=ORIENTED_EDGE('',*,*,#7583,.F.);
#9975=ORIENTED_EDGE('',*,*,#7584,.F.);
#9976=ORIENTED_EDGE('',*,*,#7585,.F.);
#9977=ORIENTED_EDGE('',*,*,#7584,.T.);
#9978=ORIENTED_EDGE('',*,*,#7586,.F.);
#9979=ORIENTED_EDGE('',*,*,#7587,.F.);
#9980=ORIENTED_EDGE('',*,*,#7588,.F.);
#9981=ORIENTED_EDGE('',*,*,#7587,.T.);
#9982=ORIENTED_EDGE('',*,*,#7589,.F.);
#9983=ORIENTED_EDGE('',*,*,#7590,.F.);
#9984=ORIENTED_EDGE('',*,*,#7591,.F.);
#9985=ORIENTED_EDGE('',*,*,#7590,.T.);
#9986=ORIENTED_EDGE('',*,*,#7592,.F.);
#9987=ORIENTED_EDGE('',*,*,#7593,.F.);
#9988=ORIENTED_EDGE('',*,*,#7594,.F.);
#9989=ORIENTED_EDGE('',*,*,#7593,.T.);
#9990=ORIENTED_EDGE('',*,*,#7595,.F.);
#9991=ORIENTED_EDGE('',*,*,#7596,.F.);
#9992=ORIENTED_EDGE('',*,*,#7597,.F.);
#9993=ORIENTED_EDGE('',*,*,#7596,.T.);
#9994=ORIENTED_EDGE('',*,*,#7598,.F.);
#9995=ORIENTED_EDGE('',*,*,#7599,.F.);
#9996=ORIENTED_EDGE('',*,*,#7600,.F.);
#9997=ORIENTED_EDGE('',*,*,#7599,.T.);
#9998=ORIENTED_EDGE('',*,*,#7601,.F.);
#9999=ORIENTED_EDGE('',*,*,#7602,.F.);
#10000=ORIENTED_EDGE('',*,*,#7603,.F.);
#10001=ORIENTED_EDGE('',*,*,#7602,.T.);
#10002=ORIENTED_EDGE('',*,*,#7604,.F.);
#10003=ORIENTED_EDGE('',*,*,#7605,.F.);
#10004=ORIENTED_EDGE('',*,*,#7606,.F.);
#10005=ORIENTED_EDGE('',*,*,#7605,.T.);
#10006=ORIENTED_EDGE('',*,*,#7607,.F.);
#10007=ORIENTED_EDGE('',*,*,#7608,.F.);
#10008=ORIENTED_EDGE('',*,*,#7609,.F.);
#10009=ORIENTED_EDGE('',*,*,#7608,.T.);
#10010=ORIENTED_EDGE('',*,*,#7610,.F.);
#10011=ORIENTED_EDGE('',*,*,#7611,.F.);
#10012=ORIENTED_EDGE('',*,*,#7612,.F.);
#10013=ORIENTED_EDGE('',*,*,#7611,.T.);
#10014=ORIENTED_EDGE('',*,*,#7613,.F.);
#10015=ORIENTED_EDGE('',*,*,#7614,.F.);
#10016=ORIENTED_EDGE('',*,*,#7615,.F.);
#10017=ORIENTED_EDGE('',*,*,#7614,.T.);
#10018=ORIENTED_EDGE('',*,*,#7616,.F.);
#10019=ORIENTED_EDGE('',*,*,#7617,.F.);
#10020=ORIENTED_EDGE('',*,*,#7618,.F.);
#10021=ORIENTED_EDGE('',*,*,#7617,.T.);
#10022=ORIENTED_EDGE('',*,*,#7619,.F.);
#10023=ORIENTED_EDGE('',*,*,#7620,.F.);
#10024=ORIENTED_EDGE('',*,*,#7621,.F.);
#10025=ORIENTED_EDGE('',*,*,#7620,.T.);
#10026=ORIENTED_EDGE('',*,*,#7622,.F.);
#10027=ORIENTED_EDGE('',*,*,#7623,.F.);
#10028=ORIENTED_EDGE('',*,*,#7624,.F.);
#10029=ORIENTED_EDGE('',*,*,#7623,.T.);
#10030=ORIENTED_EDGE('',*,*,#7625,.F.);
#10031=ORIENTED_EDGE('',*,*,#7626,.F.);
#10032=ORIENTED_EDGE('',*,*,#7627,.F.);
#10033=ORIENTED_EDGE('',*,*,#7626,.T.);
#10034=ORIENTED_EDGE('',*,*,#7628,.F.);
#10035=ORIENTED_EDGE('',*,*,#7629,.F.);
#10036=ORIENTED_EDGE('',*,*,#7630,.F.);
#10037=ORIENTED_EDGE('',*,*,#7629,.T.);
#10038=ORIENTED_EDGE('',*,*,#7631,.F.);
#10039=ORIENTED_EDGE('',*,*,#7632,.F.);
#10040=ORIENTED_EDGE('',*,*,#7633,.F.);
#10041=ORIENTED_EDGE('',*,*,#7632,.T.);
#10042=ORIENTED_EDGE('',*,*,#7634,.F.);
#10043=ORIENTED_EDGE('',*,*,#7635,.F.);
#10044=ORIENTED_EDGE('',*,*,#7636,.F.);
#10045=ORIENTED_EDGE('',*,*,#7635,.T.);
#10046=ORIENTED_EDGE('',*,*,#7637,.F.);
#10047=ORIENTED_EDGE('',*,*,#7638,.F.);
#10048=ORIENTED_EDGE('',*,*,#7639,.F.);
#10049=ORIENTED_EDGE('',*,*,#7638,.T.);
#10050=ORIENTED_EDGE('',*,*,#7640,.F.);
#10051=ORIENTED_EDGE('',*,*,#7641,.F.);
#10052=ORIENTED_EDGE('',*,*,#7642,.F.);
#10053=ORIENTED_EDGE('',*,*,#7641,.T.);
#10054=ORIENTED_EDGE('',*,*,#7643,.F.);
#10055=ORIENTED_EDGE('',*,*,#7644,.F.);
#10056=ORIENTED_EDGE('',*,*,#7645,.F.);
#10057=ORIENTED_EDGE('',*,*,#7644,.T.);
#10058=ORIENTED_EDGE('',*,*,#7646,.F.);
#10059=ORIENTED_EDGE('',*,*,#7647,.F.);
#10060=ORIENTED_EDGE('',*,*,#7648,.F.);
#10061=ORIENTED_EDGE('',*,*,#7647,.T.);
#10062=ORIENTED_EDGE('',*,*,#7649,.F.);
#10063=ORIENTED_EDGE('',*,*,#7650,.F.);
#10064=ORIENTED_EDGE('',*,*,#7651,.F.);
#10065=ORIENTED_EDGE('',*,*,#7650,.T.);
#10066=ORIENTED_EDGE('',*,*,#7652,.F.);
#10067=ORIENTED_EDGE('',*,*,#7653,.F.);
#10068=ORIENTED_EDGE('',*,*,#7654,.F.);
#10069=ORIENTED_EDGE('',*,*,#7653,.T.);
#10070=ORIENTED_EDGE('',*,*,#7655,.F.);
#10071=ORIENTED_EDGE('',*,*,#7656,.F.);
#10072=ORIENTED_EDGE('',*,*,#7657,.F.);
#10073=ORIENTED_EDGE('',*,*,#7656,.T.);
#10074=ORIENTED_EDGE('',*,*,#7658,.F.);
#10075=ORIENTED_EDGE('',*,*,#7659,.F.);
#10076=ORIENTED_EDGE('',*,*,#7660,.F.);
#10077=ORIENTED_EDGE('',*,*,#7659,.T.);
#10078=ORIENTED_EDGE('',*,*,#7661,.F.);
#10079=ORIENTED_EDGE('',*,*,#7662,.F.);
#10080=ORIENTED_EDGE('',*,*,#7663,.F.);
#10081=ORIENTED_EDGE('',*,*,#7662,.T.);
#10082=ORIENTED_EDGE('',*,*,#7664,.F.);
#10083=ORIENTED_EDGE('',*,*,#7665,.F.);
#10084=ORIENTED_EDGE('',*,*,#7666,.F.);
#10085=ORIENTED_EDGE('',*,*,#7665,.T.);
#10086=ORIENTED_EDGE('',*,*,#7667,.F.);
#10087=ORIENTED_EDGE('',*,*,#7668,.F.);
#10088=ORIENTED_EDGE('',*,*,#7669,.F.);
#10089=ORIENTED_EDGE('',*,*,#7668,.T.);
#10090=ORIENTED_EDGE('',*,*,#7670,.F.);
#10091=ORIENTED_EDGE('',*,*,#7671,.F.);
#10092=ORIENTED_EDGE('',*,*,#7672,.F.);
#10093=ORIENTED_EDGE('',*,*,#7671,.T.);
#10094=ORIENTED_EDGE('',*,*,#7673,.F.);
#10095=ORIENTED_EDGE('',*,*,#7674,.F.);
#10096=ORIENTED_EDGE('',*,*,#7675,.F.);
#10097=ORIENTED_EDGE('',*,*,#7674,.T.);
#10098=ORIENTED_EDGE('',*,*,#7676,.F.);
#10099=ORIENTED_EDGE('',*,*,#7677,.F.);
#10100=ORIENTED_EDGE('',*,*,#7678,.F.);
#10101=ORIENTED_EDGE('',*,*,#7677,.T.);
#10102=ORIENTED_EDGE('',*,*,#7679,.F.);
#10103=ORIENTED_EDGE('',*,*,#7680,.F.);
#10104=ORIENTED_EDGE('',*,*,#7681,.F.);
#10105=ORIENTED_EDGE('',*,*,#7680,.T.);
#10106=ORIENTED_EDGE('',*,*,#7682,.F.);
#10107=ORIENTED_EDGE('',*,*,#7683,.F.);
#10108=ORIENTED_EDGE('',*,*,#7684,.F.);
#10109=ORIENTED_EDGE('',*,*,#7683,.T.);
#10110=ORIENTED_EDGE('',*,*,#7685,.F.);
#10111=ORIENTED_EDGE('',*,*,#7686,.F.);
#10112=ORIENTED_EDGE('',*,*,#7687,.F.);
#10113=ORIENTED_EDGE('',*,*,#7686,.T.);
#10114=ORIENTED_EDGE('',*,*,#7688,.F.);
#10115=ORIENTED_EDGE('',*,*,#7689,.F.);
#10116=ORIENTED_EDGE('',*,*,#7690,.F.);
#10117=ORIENTED_EDGE('',*,*,#7689,.T.);
#10118=ORIENTED_EDGE('',*,*,#7691,.F.);
#10119=ORIENTED_EDGE('',*,*,#7692,.F.);
#10120=ORIENTED_EDGE('',*,*,#7693,.F.);
#10121=ORIENTED_EDGE('',*,*,#7692,.T.);
#10122=ORIENTED_EDGE('',*,*,#7694,.F.);
#10123=ORIENTED_EDGE('',*,*,#7695,.F.);
#10124=ORIENTED_EDGE('',*,*,#7696,.F.);
#10125=ORIENTED_EDGE('',*,*,#7695,.T.);
#10126=ORIENTED_EDGE('',*,*,#7697,.F.);
#10127=ORIENTED_EDGE('',*,*,#7698,.F.);
#10128=ORIENTED_EDGE('',*,*,#7699,.F.);
#10129=ORIENTED_EDGE('',*,*,#7698,.T.);
#10130=ORIENTED_EDGE('',*,*,#7700,.F.);
#10131=ORIENTED_EDGE('',*,*,#7701,.F.);
#10132=ORIENTED_EDGE('',*,*,#7702,.F.);
#10133=ORIENTED_EDGE('',*,*,#7701,.T.);
#10134=ORIENTED_EDGE('',*,*,#7703,.F.);
#10135=ORIENTED_EDGE('',*,*,#7704,.F.);
#10136=ORIENTED_EDGE('',*,*,#7705,.F.);
#10137=ORIENTED_EDGE('',*,*,#7704,.T.);
#10138=ORIENTED_EDGE('',*,*,#7706,.F.);
#10139=ORIENTED_EDGE('',*,*,#7707,.F.);
#10140=ORIENTED_EDGE('',*,*,#7708,.F.);
#10141=ORIENTED_EDGE('',*,*,#7707,.T.);
#10142=ORIENTED_EDGE('',*,*,#7709,.F.);
#10143=ORIENTED_EDGE('',*,*,#7710,.F.);
#10144=ORIENTED_EDGE('',*,*,#7711,.F.);
#10145=ORIENTED_EDGE('',*,*,#7710,.T.);
#10146=ORIENTED_EDGE('',*,*,#7712,.F.);
#10147=ORIENTED_EDGE('',*,*,#7713,.F.);
#10148=ORIENTED_EDGE('',*,*,#7714,.F.);
#10149=ORIENTED_EDGE('',*,*,#7713,.T.);
#10150=ORIENTED_EDGE('',*,*,#7715,.F.);
#10151=ORIENTED_EDGE('',*,*,#7716,.F.);
#10152=ORIENTED_EDGE('',*,*,#7717,.F.);
#10153=ORIENTED_EDGE('',*,*,#7716,.T.);
#10154=ORIENTED_EDGE('',*,*,#7718,.F.);
#10155=ORIENTED_EDGE('',*,*,#7719,.F.);
#10156=ORIENTED_EDGE('',*,*,#7720,.F.);
#10157=ORIENTED_EDGE('',*,*,#7719,.T.);
#10158=ORIENTED_EDGE('',*,*,#7721,.F.);
#10159=ORIENTED_EDGE('',*,*,#7722,.F.);
#10160=ORIENTED_EDGE('',*,*,#7723,.F.);
#10161=ORIENTED_EDGE('',*,*,#7722,.T.);
#10162=ORIENTED_EDGE('',*,*,#7724,.F.);
#10163=ORIENTED_EDGE('',*,*,#7725,.F.);
#10164=ORIENTED_EDGE('',*,*,#7726,.F.);
#10165=ORIENTED_EDGE('',*,*,#7725,.T.);
#10166=ORIENTED_EDGE('',*,*,#7727,.F.);
#10167=ORIENTED_EDGE('',*,*,#7728,.F.);
#10168=ORIENTED_EDGE('',*,*,#7729,.F.);
#10169=ORIENTED_EDGE('',*,*,#7728,.T.);
#10170=ORIENTED_EDGE('',*,*,#7730,.F.);
#10171=ORIENTED_EDGE('',*,*,#7731,.F.);
#10172=ORIENTED_EDGE('',*,*,#7732,.F.);
#10173=ORIENTED_EDGE('',*,*,#7731,.T.);
#10174=ORIENTED_EDGE('',*,*,#7733,.F.);
#10175=ORIENTED_EDGE('',*,*,#7734,.F.);
#10176=ORIENTED_EDGE('',*,*,#7735,.F.);
#10177=ORIENTED_EDGE('',*,*,#7734,.T.);
#10178=ORIENTED_EDGE('',*,*,#7736,.F.);
#10179=ORIENTED_EDGE('',*,*,#7737,.F.);
#10180=ORIENTED_EDGE('',*,*,#7738,.F.);
#10181=ORIENTED_EDGE('',*,*,#7737,.T.);
#10182=ORIENTED_EDGE('',*,*,#7739,.F.);
#10183=ORIENTED_EDGE('',*,*,#7740,.F.);
#10184=ORIENTED_EDGE('',*,*,#7741,.F.);
#10185=ORIENTED_EDGE('',*,*,#7740,.T.);
#10186=ORIENTED_EDGE('',*,*,#7742,.F.);
#10187=ORIENTED_EDGE('',*,*,#7743,.F.);
#10188=ORIENTED_EDGE('',*,*,#7744,.F.);
#10189=ORIENTED_EDGE('',*,*,#7743,.T.);
#10190=ORIENTED_EDGE('',*,*,#7745,.F.);
#10191=ORIENTED_EDGE('',*,*,#7746,.F.);
#10192=ORIENTED_EDGE('',*,*,#7747,.F.);
#10193=ORIENTED_EDGE('',*,*,#7746,.T.);
#10194=ORIENTED_EDGE('',*,*,#7748,.F.);
#10195=ORIENTED_EDGE('',*,*,#7749,.F.);
#10196=ORIENTED_EDGE('',*,*,#7750,.F.);
#10197=ORIENTED_EDGE('',*,*,#7749,.T.);
#10198=ORIENTED_EDGE('',*,*,#7751,.F.);
#10199=ORIENTED_EDGE('',*,*,#7752,.F.);
#10200=ORIENTED_EDGE('',*,*,#7753,.F.);
#10201=ORIENTED_EDGE('',*,*,#7752,.T.);
#10202=ORIENTED_EDGE('',*,*,#7754,.F.);
#10203=ORIENTED_EDGE('',*,*,#7755,.F.);
#10204=ORIENTED_EDGE('',*,*,#7756,.F.);
#10205=ORIENTED_EDGE('',*,*,#7755,.T.);
#10206=ORIENTED_EDGE('',*,*,#7757,.F.);
#10207=ORIENTED_EDGE('',*,*,#7758,.F.);
#10208=ORIENTED_EDGE('',*,*,#7759,.F.);
#10209=ORIENTED_EDGE('',*,*,#7758,.T.);
#10210=ORIENTED_EDGE('',*,*,#7760,.F.);
#10211=ORIENTED_EDGE('',*,*,#7761,.F.);
#10212=ORIENTED_EDGE('',*,*,#7762,.F.);
#10213=ORIENTED_EDGE('',*,*,#7761,.T.);
#10214=ORIENTED_EDGE('',*,*,#7763,.F.);
#10215=ORIENTED_EDGE('',*,*,#7764,.F.);
#10216=ORIENTED_EDGE('',*,*,#7765,.F.);
#10217=ORIENTED_EDGE('',*,*,#7764,.T.);
#10218=ORIENTED_EDGE('',*,*,#7766,.F.);
#10219=ORIENTED_EDGE('',*,*,#7767,.F.);
#10220=ORIENTED_EDGE('',*,*,#7768,.F.);
#10221=ORIENTED_EDGE('',*,*,#7767,.T.);
#10222=ORIENTED_EDGE('',*,*,#7769,.F.);
#10223=ORIENTED_EDGE('',*,*,#7770,.F.);
#10224=ORIENTED_EDGE('',*,*,#7771,.F.);
#10225=ORIENTED_EDGE('',*,*,#7770,.T.);
#10226=ORIENTED_EDGE('',*,*,#7772,.F.);
#10227=ORIENTED_EDGE('',*,*,#7773,.F.);
#10228=ORIENTED_EDGE('',*,*,#7774,.F.);
#10229=ORIENTED_EDGE('',*,*,#7773,.T.);
#10230=ORIENTED_EDGE('',*,*,#7775,.F.);
#10231=ORIENTED_EDGE('',*,*,#7776,.F.);
#10232=ORIENTED_EDGE('',*,*,#7777,.F.);
#10233=ORIENTED_EDGE('',*,*,#7776,.T.);
#10234=ORIENTED_EDGE('',*,*,#7778,.F.);
#10235=ORIENTED_EDGE('',*,*,#7779,.F.);
#10236=ORIENTED_EDGE('',*,*,#7780,.F.);
#10237=ORIENTED_EDGE('',*,*,#7779,.T.);
#10238=ORIENTED_EDGE('',*,*,#7781,.F.);
#10239=ORIENTED_EDGE('',*,*,#7782,.F.);
#10240=ORIENTED_EDGE('',*,*,#7783,.F.);
#10241=ORIENTED_EDGE('',*,*,#7782,.T.);
#10242=ORIENTED_EDGE('',*,*,#7784,.F.);
#10243=ORIENTED_EDGE('',*,*,#7785,.F.);
#10244=ORIENTED_EDGE('',*,*,#7786,.F.);
#10245=ORIENTED_EDGE('',*,*,#7785,.T.);
#10246=ORIENTED_EDGE('',*,*,#7787,.F.);
#10247=ORIENTED_EDGE('',*,*,#7788,.F.);
#10248=ORIENTED_EDGE('',*,*,#7789,.F.);
#10249=ORIENTED_EDGE('',*,*,#7788,.T.);
#10250=ORIENTED_EDGE('',*,*,#7790,.F.);
#10251=ORIENTED_EDGE('',*,*,#7791,.F.);
#10252=ORIENTED_EDGE('',*,*,#7792,.F.);
#10253=ORIENTED_EDGE('',*,*,#7791,.T.);
#10254=ORIENTED_EDGE('',*,*,#7793,.F.);
#10255=ORIENTED_EDGE('',*,*,#7794,.F.);
#10256=ORIENTED_EDGE('',*,*,#7795,.F.);
#10257=ORIENTED_EDGE('',*,*,#7794,.T.);
#10258=ORIENTED_EDGE('',*,*,#7796,.F.);
#10259=ORIENTED_EDGE('',*,*,#7797,.F.);
#10260=ORIENTED_EDGE('',*,*,#7798,.F.);
#10261=ORIENTED_EDGE('',*,*,#7797,.T.);
#10262=ORIENTED_EDGE('',*,*,#7799,.F.);
#10263=ORIENTED_EDGE('',*,*,#7800,.F.);
#10264=ORIENTED_EDGE('',*,*,#7801,.F.);
#10265=ORIENTED_EDGE('',*,*,#7800,.T.);
#10266=ORIENTED_EDGE('',*,*,#7802,.F.);
#10267=ORIENTED_EDGE('',*,*,#7803,.F.);
#10268=ORIENTED_EDGE('',*,*,#7804,.F.);
#10269=ORIENTED_EDGE('',*,*,#7803,.T.);
#10270=ORIENTED_EDGE('',*,*,#7805,.F.);
#10271=ORIENTED_EDGE('',*,*,#7806,.F.);
#10272=ORIENTED_EDGE('',*,*,#7807,.F.);
#10273=ORIENTED_EDGE('',*,*,#7806,.T.);
#10274=ORIENTED_EDGE('',*,*,#7808,.F.);
#10275=ORIENTED_EDGE('',*,*,#7809,.F.);
#10276=ORIENTED_EDGE('',*,*,#7810,.F.);
#10277=ORIENTED_EDGE('',*,*,#7809,.T.);
#10278=ORIENTED_EDGE('',*,*,#7811,.F.);
#10279=ORIENTED_EDGE('',*,*,#7812,.F.);
#10280=ORIENTED_EDGE('',*,*,#7813,.F.);
#10281=ORIENTED_EDGE('',*,*,#7812,.T.);
#10282=ORIENTED_EDGE('',*,*,#7814,.F.);
#10283=ORIENTED_EDGE('',*,*,#7815,.F.);
#10284=ORIENTED_EDGE('',*,*,#7816,.F.);
#10285=ORIENTED_EDGE('',*,*,#7815,.T.);
#10286=ORIENTED_EDGE('',*,*,#7817,.F.);
#10287=ORIENTED_EDGE('',*,*,#7818,.F.);
#10288=ORIENTED_EDGE('',*,*,#7819,.F.);
#10289=ORIENTED_EDGE('',*,*,#7818,.T.);
#10290=ORIENTED_EDGE('',*,*,#7820,.F.);
#10291=ORIENTED_EDGE('',*,*,#7821,.F.);
#10292=ORIENTED_EDGE('',*,*,#7822,.F.);
#10293=ORIENTED_EDGE('',*,*,#7821,.T.);
#10294=ORIENTED_EDGE('',*,*,#7823,.F.);
#10295=ORIENTED_EDGE('',*,*,#7824,.F.);
#10296=ORIENTED_EDGE('',*,*,#7825,.F.);
#10297=ORIENTED_EDGE('',*,*,#7824,.T.);
#10298=ORIENTED_EDGE('',*,*,#7826,.F.);
#10299=ORIENTED_EDGE('',*,*,#7827,.F.);
#10300=ORIENTED_EDGE('',*,*,#7828,.F.);
#10301=ORIENTED_EDGE('',*,*,#7827,.T.);
#10302=ORIENTED_EDGE('',*,*,#7829,.F.);
#10303=ORIENTED_EDGE('',*,*,#7830,.F.);
#10304=ORIENTED_EDGE('',*,*,#7831,.F.);
#10305=ORIENTED_EDGE('',*,*,#7830,.T.);
#10306=ORIENTED_EDGE('',*,*,#7832,.F.);
#10307=ORIENTED_EDGE('',*,*,#7833,.F.);
#10308=ORIENTED_EDGE('',*,*,#7834,.F.);
#10309=ORIENTED_EDGE('',*,*,#7833,.T.);
#10310=ORIENTED_EDGE('',*,*,#7835,.F.);
#10311=ORIENTED_EDGE('',*,*,#7836,.F.);
#10312=ORIENTED_EDGE('',*,*,#7837,.F.);
#10313=ORIENTED_EDGE('',*,*,#7836,.T.);
#10314=ORIENTED_EDGE('',*,*,#7838,.F.);
#10315=ORIENTED_EDGE('',*,*,#7839,.F.);
#10316=ORIENTED_EDGE('',*,*,#7840,.F.);
#10317=ORIENTED_EDGE('',*,*,#7839,.T.);
#10318=ORIENTED_EDGE('',*,*,#7841,.F.);
#10319=ORIENTED_EDGE('',*,*,#7842,.F.);
#10320=ORIENTED_EDGE('',*,*,#7843,.F.);
#10321=ORIENTED_EDGE('',*,*,#7842,.T.);
#10322=ORIENTED_EDGE('',*,*,#7844,.F.);
#10323=ORIENTED_EDGE('',*,*,#7845,.F.);
#10324=ORIENTED_EDGE('',*,*,#7846,.F.);
#10325=ORIENTED_EDGE('',*,*,#7845,.T.);
#10326=ORIENTED_EDGE('',*,*,#7847,.F.);
#10327=ORIENTED_EDGE('',*,*,#7848,.F.);
#10328=ORIENTED_EDGE('',*,*,#7849,.F.);
#10329=ORIENTED_EDGE('',*,*,#7848,.T.);
#10330=ORIENTED_EDGE('',*,*,#7850,.F.);
#10331=ORIENTED_EDGE('',*,*,#7851,.F.);
#10332=ORIENTED_EDGE('',*,*,#7852,.F.);
#10333=ORIENTED_EDGE('',*,*,#7851,.T.);
#10334=ORIENTED_EDGE('',*,*,#7853,.F.);
#10335=ORIENTED_EDGE('',*,*,#7854,.F.);
#10336=ORIENTED_EDGE('',*,*,#7855,.F.);
#10337=ORIENTED_EDGE('',*,*,#7854,.T.);
#10338=ORIENTED_EDGE('',*,*,#7856,.F.);
#10339=ORIENTED_EDGE('',*,*,#7857,.F.);
#10340=ORIENTED_EDGE('',*,*,#7858,.F.);
#10341=ORIENTED_EDGE('',*,*,#7857,.T.);
#10342=ORIENTED_EDGE('',*,*,#7859,.F.);
#10343=ORIENTED_EDGE('',*,*,#7860,.F.);
#10344=ORIENTED_EDGE('',*,*,#7861,.F.);
#10345=ORIENTED_EDGE('',*,*,#7860,.T.);
#10346=ORIENTED_EDGE('',*,*,#7862,.F.);
#10347=ORIENTED_EDGE('',*,*,#7863,.F.);
#10348=ORIENTED_EDGE('',*,*,#7864,.F.);
#10349=ORIENTED_EDGE('',*,*,#7863,.T.);
#10350=ORIENTED_EDGE('',*,*,#7865,.F.);
#10351=ORIENTED_EDGE('',*,*,#7866,.F.);
#10352=ORIENTED_EDGE('',*,*,#7867,.F.);
#10353=ORIENTED_EDGE('',*,*,#7866,.T.);
#10354=ORIENTED_EDGE('',*,*,#7868,.F.);
#10355=ORIENTED_EDGE('',*,*,#7869,.F.);
#10356=ORIENTED_EDGE('',*,*,#7870,.F.);
#10357=ORIENTED_EDGE('',*,*,#7869,.T.);
#10358=ORIENTED_EDGE('',*,*,#7871,.F.);
#10359=ORIENTED_EDGE('',*,*,#7872,.F.);
#10360=ORIENTED_EDGE('',*,*,#7873,.F.);
#10361=ORIENTED_EDGE('',*,*,#7872,.T.);
#10362=ORIENTED_EDGE('',*,*,#7874,.F.);
#10363=ORIENTED_EDGE('',*,*,#7875,.F.);
#10364=ORIENTED_EDGE('',*,*,#7876,.F.);
#10365=ORIENTED_EDGE('',*,*,#7875,.T.);
#10366=ORIENTED_EDGE('',*,*,#7877,.F.);
#10367=ORIENTED_EDGE('',*,*,#7878,.F.);
#10368=ORIENTED_EDGE('',*,*,#7879,.F.);
#10369=ORIENTED_EDGE('',*,*,#7878,.T.);
#10370=ORIENTED_EDGE('',*,*,#7880,.F.);
#10371=ORIENTED_EDGE('',*,*,#7881,.F.);
#10372=ORIENTED_EDGE('',*,*,#7882,.F.);
#10373=ORIENTED_EDGE('',*,*,#7881,.T.);
#10374=ORIENTED_EDGE('',*,*,#7883,.F.);
#10375=ORIENTED_EDGE('',*,*,#7394,.F.);
#10376=ORIENTED_EDGE('',*,*,#7883,.T.);
#10377=ORIENTED_EDGE('',*,*,#7880,.T.);
#10378=ORIENTED_EDGE('',*,*,#7877,.T.);
#10379=ORIENTED_EDGE('',*,*,#7874,.T.);
#10380=ORIENTED_EDGE('',*,*,#7871,.T.);
#10381=ORIENTED_EDGE('',*,*,#7868,.T.);
#10382=ORIENTED_EDGE('',*,*,#7865,.T.);
#10383=ORIENTED_EDGE('',*,*,#7862,.T.);
#10384=ORIENTED_EDGE('',*,*,#7859,.T.);
#10385=ORIENTED_EDGE('',*,*,#7856,.T.);
#10386=ORIENTED_EDGE('',*,*,#7853,.T.);
#10387=ORIENTED_EDGE('',*,*,#7850,.T.);
#10388=ORIENTED_EDGE('',*,*,#7847,.T.);
#10389=ORIENTED_EDGE('',*,*,#7844,.T.);
#10390=ORIENTED_EDGE('',*,*,#7841,.T.);
#10391=ORIENTED_EDGE('',*,*,#7838,.T.);
#10392=ORIENTED_EDGE('',*,*,#7835,.T.);
#10393=ORIENTED_EDGE('',*,*,#7832,.T.);
#10394=ORIENTED_EDGE('',*,*,#7829,.T.);
#10395=ORIENTED_EDGE('',*,*,#7826,.T.);
#10396=ORIENTED_EDGE('',*,*,#7823,.T.);
#10397=ORIENTED_EDGE('',*,*,#7820,.T.);
#10398=ORIENTED_EDGE('',*,*,#7817,.T.);
#10399=ORIENTED_EDGE('',*,*,#7814,.T.);
#10400=ORIENTED_EDGE('',*,*,#7811,.T.);
#10401=ORIENTED_EDGE('',*,*,#7808,.T.);
#10402=ORIENTED_EDGE('',*,*,#7805,.T.);
#10403=ORIENTED_EDGE('',*,*,#7802,.T.);
#10404=ORIENTED_EDGE('',*,*,#7799,.T.);
#10405=ORIENTED_EDGE('',*,*,#7796,.T.);
#10406=ORIENTED_EDGE('',*,*,#7793,.T.);
#10407=ORIENTED_EDGE('',*,*,#7790,.T.);
#10408=ORIENTED_EDGE('',*,*,#7787,.T.);
#10409=ORIENTED_EDGE('',*,*,#7784,.T.);
#10410=ORIENTED_EDGE('',*,*,#7781,.T.);
#10411=ORIENTED_EDGE('',*,*,#7778,.T.);
#10412=ORIENTED_EDGE('',*,*,#7775,.T.);
#10413=ORIENTED_EDGE('',*,*,#7772,.T.);
#10414=ORIENTED_EDGE('',*,*,#7769,.T.);
#10415=ORIENTED_EDGE('',*,*,#7766,.T.);
#10416=ORIENTED_EDGE('',*,*,#7763,.T.);
#10417=ORIENTED_EDGE('',*,*,#7760,.T.);
#10418=ORIENTED_EDGE('',*,*,#7757,.T.);
#10419=ORIENTED_EDGE('',*,*,#7754,.T.);
#10420=ORIENTED_EDGE('',*,*,#7751,.T.);
#10421=ORIENTED_EDGE('',*,*,#7748,.T.);
#10422=ORIENTED_EDGE('',*,*,#7745,.T.);
#10423=ORIENTED_EDGE('',*,*,#7742,.T.);
#10424=ORIENTED_EDGE('',*,*,#7739,.T.);
#10425=ORIENTED_EDGE('',*,*,#7736,.T.);
#10426=ORIENTED_EDGE('',*,*,#7733,.T.);
#10427=ORIENTED_EDGE('',*,*,#7730,.T.);
#10428=ORIENTED_EDGE('',*,*,#7727,.T.);
#10429=ORIENTED_EDGE('',*,*,#7724,.T.);
#10430=ORIENTED_EDGE('',*,*,#7721,.T.);
#10431=ORIENTED_EDGE('',*,*,#7718,.T.);
#10432=ORIENTED_EDGE('',*,*,#7715,.T.);
#10433=ORIENTED_EDGE('',*,*,#7712,.T.);
#10434=ORIENTED_EDGE('',*,*,#7709,.T.);
#10435=ORIENTED_EDGE('',*,*,#7706,.T.);
#10436=ORIENTED_EDGE('',*,*,#7703,.T.);
#10437=ORIENTED_EDGE('',*,*,#7700,.T.);
#10438=ORIENTED_EDGE('',*,*,#7697,.T.);
#10439=ORIENTED_EDGE('',*,*,#7694,.T.);
#10440=ORIENTED_EDGE('',*,*,#7691,.T.);
#10441=ORIENTED_EDGE('',*,*,#7688,.T.);
#10442=ORIENTED_EDGE('',*,*,#7685,.T.);
#10443=ORIENTED_EDGE('',*,*,#7682,.T.);
#10444=ORIENTED_EDGE('',*,*,#7679,.T.);
#10445=ORIENTED_EDGE('',*,*,#7676,.T.);
#10446=ORIENTED_EDGE('',*,*,#7673,.T.);
#10447=ORIENTED_EDGE('',*,*,#7670,.T.);
#10448=ORIENTED_EDGE('',*,*,#7667,.T.);
#10449=ORIENTED_EDGE('',*,*,#7664,.T.);
#10450=ORIENTED_EDGE('',*,*,#7661,.T.);
#10451=ORIENTED_EDGE('',*,*,#7658,.T.);
#10452=ORIENTED_EDGE('',*,*,#7655,.T.);
#10453=ORIENTED_EDGE('',*,*,#7652,.T.);
#10454=ORIENTED_EDGE('',*,*,#7649,.T.);
#10455=ORIENTED_EDGE('',*,*,#7646,.T.);
#10456=ORIENTED_EDGE('',*,*,#7643,.T.);
#10457=ORIENTED_EDGE('',*,*,#7640,.T.);
#10458=ORIENTED_EDGE('',*,*,#7637,.T.);
#10459=ORIENTED_EDGE('',*,*,#7634,.T.);
#10460=ORIENTED_EDGE('',*,*,#7631,.T.);
#10461=ORIENTED_EDGE('',*,*,#7628,.T.);
#10462=ORIENTED_EDGE('',*,*,#7625,.T.);
#10463=ORIENTED_EDGE('',*,*,#7622,.T.);
#10464=ORIENTED_EDGE('',*,*,#7619,.T.);
#10465=ORIENTED_EDGE('',*,*,#7616,.T.);
#10466=ORIENTED_EDGE('',*,*,#7613,.T.);
#10467=ORIENTED_EDGE('',*,*,#7610,.T.);
#10468=ORIENTED_EDGE('',*,*,#7607,.T.);
#10469=ORIENTED_EDGE('',*,*,#7604,.T.);
#10470=ORIENTED_EDGE('',*,*,#7601,.T.);
#10471=ORIENTED_EDGE('',*,*,#7598,.T.);
#10472=ORIENTED_EDGE('',*,*,#7595,.T.);
#10473=ORIENTED_EDGE('',*,*,#7592,.T.);
#10474=ORIENTED_EDGE('',*,*,#7589,.T.);
#10475=ORIENTED_EDGE('',*,*,#7586,.T.);
#10476=ORIENTED_EDGE('',*,*,#7583,.T.);
#10477=ORIENTED_EDGE('',*,*,#7580,.T.);
#10478=ORIENTED_EDGE('',*,*,#7577,.T.);
#10479=ORIENTED_EDGE('',*,*,#7574,.T.);
#10480=ORIENTED_EDGE('',*,*,#7571,.T.);
#10481=ORIENTED_EDGE('',*,*,#7568,.T.);
#10482=ORIENTED_EDGE('',*,*,#7565,.T.);
#10483=ORIENTED_EDGE('',*,*,#7562,.T.);
#10484=ORIENTED_EDGE('',*,*,#7559,.T.);
#10485=ORIENTED_EDGE('',*,*,#7556,.T.);
#10486=ORIENTED_EDGE('',*,*,#7553,.T.);
#10487=ORIENTED_EDGE('',*,*,#7550,.T.);
#10488=ORIENTED_EDGE('',*,*,#7547,.T.);
#10489=ORIENTED_EDGE('',*,*,#7544,.T.);
#10490=ORIENTED_EDGE('',*,*,#7541,.T.);
#10491=ORIENTED_EDGE('',*,*,#7538,.T.);
#10492=ORIENTED_EDGE('',*,*,#7535,.T.);
#10493=ORIENTED_EDGE('',*,*,#7532,.T.);
#10494=ORIENTED_EDGE('',*,*,#7529,.T.);
#10495=ORIENTED_EDGE('',*,*,#7526,.T.);
#10496=ORIENTED_EDGE('',*,*,#7523,.T.);
#10497=ORIENTED_EDGE('',*,*,#7520,.T.);
#10498=ORIENTED_EDGE('',*,*,#7517,.T.);
#10499=ORIENTED_EDGE('',*,*,#7514,.T.);
#10500=ORIENTED_EDGE('',*,*,#7511,.T.);
#10501=ORIENTED_EDGE('',*,*,#7508,.T.);
#10502=ORIENTED_EDGE('',*,*,#7505,.T.);
#10503=ORIENTED_EDGE('',*,*,#7502,.T.);
#10504=ORIENTED_EDGE('',*,*,#7499,.T.);
#10505=ORIENTED_EDGE('',*,*,#7496,.T.);
#10506=ORIENTED_EDGE('',*,*,#7493,.T.);
#10507=ORIENTED_EDGE('',*,*,#7490,.T.);
#10508=ORIENTED_EDGE('',*,*,#7487,.T.);
#10509=ORIENTED_EDGE('',*,*,#7484,.T.);
#10510=ORIENTED_EDGE('',*,*,#7481,.T.);
#10511=ORIENTED_EDGE('',*,*,#7478,.T.);
#10512=ORIENTED_EDGE('',*,*,#7475,.T.);
#10513=ORIENTED_EDGE('',*,*,#7472,.T.);
#10514=ORIENTED_EDGE('',*,*,#7469,.T.);
#10515=ORIENTED_EDGE('',*,*,#7466,.T.);
#10516=ORIENTED_EDGE('',*,*,#7463,.T.);
#10517=ORIENTED_EDGE('',*,*,#7460,.T.);
#10518=ORIENTED_EDGE('',*,*,#7457,.T.);
#10519=ORIENTED_EDGE('',*,*,#7454,.T.);
#10520=ORIENTED_EDGE('',*,*,#7451,.T.);
#10521=ORIENTED_EDGE('',*,*,#7448,.T.);
#10522=ORIENTED_EDGE('',*,*,#7445,.T.);
#10523=ORIENTED_EDGE('',*,*,#7442,.T.);
#10524=ORIENTED_EDGE('',*,*,#7439,.T.);
#10525=ORIENTED_EDGE('',*,*,#7436,.T.);
#10526=ORIENTED_EDGE('',*,*,#7433,.T.);
#10527=ORIENTED_EDGE('',*,*,#7430,.T.);
#10528=ORIENTED_EDGE('',*,*,#7427,.T.);
#10529=ORIENTED_EDGE('',*,*,#7424,.T.);
#10530=ORIENTED_EDGE('',*,*,#7421,.T.);
#10531=ORIENTED_EDGE('',*,*,#7418,.T.);
#10532=ORIENTED_EDGE('',*,*,#7415,.T.);
#10533=ORIENTED_EDGE('',*,*,#7412,.T.);
#10534=ORIENTED_EDGE('',*,*,#7409,.T.);
#10535=ORIENTED_EDGE('',*,*,#7406,.T.);
#10536=ORIENTED_EDGE('',*,*,#7403,.T.);
#10537=ORIENTED_EDGE('',*,*,#7398,.T.);
#10538=ORIENTED_EDGE('',*,*,#7390,.T.);
#10539=ORIENTED_EDGE('',*,*,#7395,.T.);
#10540=ORIENTED_EDGE('',*,*,#7882,.T.);
#10541=ORIENTED_EDGE('',*,*,#7393,.T.);
#10542=ORIENTED_EDGE('',*,*,#7386,.T.);
#10543=ORIENTED_EDGE('',*,*,#7400,.T.);
#10544=ORIENTED_EDGE('',*,*,#7402,.T.);
#10545=ORIENTED_EDGE('',*,*,#7405,.T.);
#10546=ORIENTED_EDGE('',*,*,#7408,.T.);
#10547=ORIENTED_EDGE('',*,*,#7411,.T.);
#10548=ORIENTED_EDGE('',*,*,#7414,.T.);
#10549=ORIENTED_EDGE('',*,*,#7417,.T.);
#10550=ORIENTED_EDGE('',*,*,#7420,.T.);
#10551=ORIENTED_EDGE('',*,*,#7423,.T.);
#10552=ORIENTED_EDGE('',*,*,#7426,.T.);
#10553=ORIENTED_EDGE('',*,*,#7429,.T.);
#10554=ORIENTED_EDGE('',*,*,#7432,.T.);
#10555=ORIENTED_EDGE('',*,*,#7435,.T.);
#10556=ORIENTED_EDGE('',*,*,#7438,.T.);
#10557=ORIENTED_EDGE('',*,*,#7441,.T.);
#10558=ORIENTED_EDGE('',*,*,#7444,.T.);
#10559=ORIENTED_EDGE('',*,*,#7447,.T.);
#10560=ORIENTED_EDGE('',*,*,#7450,.T.);
#10561=ORIENTED_EDGE('',*,*,#7453,.T.);
#10562=ORIENTED_EDGE('',*,*,#7456,.T.);
#10563=ORIENTED_EDGE('',*,*,#7459,.T.);
#10564=ORIENTED_EDGE('',*,*,#7462,.T.);
#10565=ORIENTED_EDGE('',*,*,#7465,.T.);
#10566=ORIENTED_EDGE('',*,*,#7468,.T.);
#10567=ORIENTED_EDGE('',*,*,#7471,.T.);
#10568=ORIENTED_EDGE('',*,*,#7474,.T.);
#10569=ORIENTED_EDGE('',*,*,#7477,.T.);
#10570=ORIENTED_EDGE('',*,*,#7480,.T.);
#10571=ORIENTED_EDGE('',*,*,#7483,.T.);
#10572=ORIENTED_EDGE('',*,*,#7486,.T.);
#10573=ORIENTED_EDGE('',*,*,#7489,.T.);
#10574=ORIENTED_EDGE('',*,*,#7492,.T.);
#10575=ORIENTED_EDGE('',*,*,#7495,.T.);
#10576=ORIENTED_EDGE('',*,*,#7498,.T.);
#10577=ORIENTED_EDGE('',*,*,#7501,.T.);
#10578=ORIENTED_EDGE('',*,*,#7504,.T.);
#10579=ORIENTED_EDGE('',*,*,#7507,.T.);
#10580=ORIENTED_EDGE('',*,*,#7510,.T.);
#10581=ORIENTED_EDGE('',*,*,#7513,.T.);
#10582=ORIENTED_EDGE('',*,*,#7516,.T.);
#10583=ORIENTED_EDGE('',*,*,#7519,.T.);
#10584=ORIENTED_EDGE('',*,*,#7522,.T.);
#10585=ORIENTED_EDGE('',*,*,#7525,.T.);
#10586=ORIENTED_EDGE('',*,*,#7528,.T.);
#10587=ORIENTED_EDGE('',*,*,#7531,.T.);
#10588=ORIENTED_EDGE('',*,*,#7534,.T.);
#10589=ORIENTED_EDGE('',*,*,#7537,.T.);
#10590=ORIENTED_EDGE('',*,*,#7540,.T.);
#10591=ORIENTED_EDGE('',*,*,#7543,.T.);
#10592=ORIENTED_EDGE('',*,*,#7546,.T.);
#10593=ORIENTED_EDGE('',*,*,#7549,.T.);
#10594=ORIENTED_EDGE('',*,*,#7552,.T.);
#10595=ORIENTED_EDGE('',*,*,#7555,.T.);
#10596=ORIENTED_EDGE('',*,*,#7558,.T.);
#10597=ORIENTED_EDGE('',*,*,#7561,.T.);
#10598=ORIENTED_EDGE('',*,*,#7564,.T.);
#10599=ORIENTED_EDGE('',*,*,#7567,.T.);
#10600=ORIENTED_EDGE('',*,*,#7570,.T.);
#10601=ORIENTED_EDGE('',*,*,#7573,.T.);
#10602=ORIENTED_EDGE('',*,*,#7576,.T.);
#10603=ORIENTED_EDGE('',*,*,#7579,.T.);
#10604=ORIENTED_EDGE('',*,*,#7582,.T.);
#10605=ORIENTED_EDGE('',*,*,#7585,.T.);
#10606=ORIENTED_EDGE('',*,*,#7588,.T.);
#10607=ORIENTED_EDGE('',*,*,#7591,.T.);
#10608=ORIENTED_EDGE('',*,*,#7594,.T.);
#10609=ORIENTED_EDGE('',*,*,#7597,.T.);
#10610=ORIENTED_EDGE('',*,*,#7600,.T.);
#10611=ORIENTED_EDGE('',*,*,#7603,.T.);
#10612=ORIENTED_EDGE('',*,*,#7606,.T.);
#10613=ORIENTED_EDGE('',*,*,#7609,.T.);
#10614=ORIENTED_EDGE('',*,*,#7612,.T.);
#10615=ORIENTED_EDGE('',*,*,#7615,.T.);
#10616=ORIENTED_EDGE('',*,*,#7618,.T.);
#10617=ORIENTED_EDGE('',*,*,#7621,.T.);
#10618=ORIENTED_EDGE('',*,*,#7624,.T.);
#10619=ORIENTED_EDGE('',*,*,#7627,.T.);
#10620=ORIENTED_EDGE('',*,*,#7630,.T.);
#10621=ORIENTED_EDGE('',*,*,#7633,.T.);
#10622=ORIENTED_EDGE('',*,*,#7636,.T.);
#10623=ORIENTED_EDGE('',*,*,#7639,.T.);
#10624=ORIENTED_EDGE('',*,*,#7642,.T.);
#10625=ORIENTED_EDGE('',*,*,#7645,.T.);
#10626=ORIENTED_EDGE('',*,*,#7648,.T.);
#10627=ORIENTED_EDGE('',*,*,#7651,.T.);
#10628=ORIENTED_EDGE('',*,*,#7654,.T.);
#10629=ORIENTED_EDGE('',*,*,#7657,.T.);
#10630=ORIENTED_EDGE('',*,*,#7660,.T.);
#10631=ORIENTED_EDGE('',*,*,#7663,.T.);
#10632=ORIENTED_EDGE('',*,*,#7666,.T.);
#10633=ORIENTED_EDGE('',*,*,#7669,.T.);
#10634=ORIENTED_EDGE('',*,*,#7672,.T.);
#10635=ORIENTED_EDGE('',*,*,#7675,.T.);
#10636=ORIENTED_EDGE('',*,*,#7678,.T.);
#10637=ORIENTED_EDGE('',*,*,#7681,.T.);
#10638=ORIENTED_EDGE('',*,*,#7684,.T.);
#10639=ORIENTED_EDGE('',*,*,#7687,.T.);
#10640=ORIENTED_EDGE('',*,*,#7690,.T.);
#10641=ORIENTED_EDGE('',*,*,#7693,.T.);
#10642=ORIENTED_EDGE('',*,*,#7696,.T.);
#10643=ORIENTED_EDGE('',*,*,#7699,.T.);
#10644=ORIENTED_EDGE('',*,*,#7702,.T.);
#10645=ORIENTED_EDGE('',*,*,#7705,.T.);
#10646=ORIENTED_EDGE('',*,*,#7708,.T.);
#10647=ORIENTED_EDGE('',*,*,#7711,.T.);
#10648=ORIENTED_EDGE('',*,*,#7714,.T.);
#10649=ORIENTED_EDGE('',*,*,#7717,.T.);
#10650=ORIENTED_EDGE('',*,*,#7720,.T.);
#10651=ORIENTED_EDGE('',*,*,#7723,.T.);
#10652=ORIENTED_EDGE('',*,*,#7726,.T.);
#10653=ORIENTED_EDGE('',*,*,#7729,.T.);
#10654=ORIENTED_EDGE('',*,*,#7732,.T.);
#10655=ORIENTED_EDGE('',*,*,#7735,.T.);
#10656=ORIENTED_EDGE('',*,*,#7738,.T.);
#10657=ORIENTED_EDGE('',*,*,#7741,.T.);
#10658=ORIENTED_EDGE('',*,*,#7744,.T.);
#10659=ORIENTED_EDGE('',*,*,#7747,.T.);
#10660=ORIENTED_EDGE('',*,*,#7750,.T.);
#10661=ORIENTED_EDGE('',*,*,#7753,.T.);
#10662=ORIENTED_EDGE('',*,*,#7756,.T.);
#10663=ORIENTED_EDGE('',*,*,#7759,.T.);
#10664=ORIENTED_EDGE('',*,*,#7762,.T.);
#10665=ORIENTED_EDGE('',*,*,#7765,.T.);
#10666=ORIENTED_EDGE('',*,*,#7768,.T.);
#10667=ORIENTED_EDGE('',*,*,#7771,.T.);
#10668=ORIENTED_EDGE('',*,*,#7774,.T.);
#10669=ORIENTED_EDGE('',*,*,#7777,.T.);
#10670=ORIENTED_EDGE('',*,*,#7780,.T.);
#10671=ORIENTED_EDGE('',*,*,#7783,.T.);
#10672=ORIENTED_EDGE('',*,*,#7786,.T.);
#10673=ORIENTED_EDGE('',*,*,#7789,.T.);
#10674=ORIENTED_EDGE('',*,*,#7792,.T.);
#10675=ORIENTED_EDGE('',*,*,#7795,.T.);
#10676=ORIENTED_EDGE('',*,*,#7798,.T.);
#10677=ORIENTED_EDGE('',*,*,#7801,.T.);
#10678=ORIENTED_EDGE('',*,*,#7804,.T.);
#10679=ORIENTED_EDGE('',*,*,#7807,.T.);
#10680=ORIENTED_EDGE('',*,*,#7810,.T.);
#10681=ORIENTED_EDGE('',*,*,#7813,.T.);
#10682=ORIENTED_EDGE('',*,*,#7816,.T.);
#10683=ORIENTED_EDGE('',*,*,#7819,.T.);
#10684=ORIENTED_EDGE('',*,*,#7822,.T.);
#10685=ORIENTED_EDGE('',*,*,#7825,.T.);
#10686=ORIENTED_EDGE('',*,*,#7828,.T.);
#10687=ORIENTED_EDGE('',*,*,#7831,.T.);
#10688=ORIENTED_EDGE('',*,*,#7834,.T.);
#10689=ORIENTED_EDGE('',*,*,#7837,.T.);
#10690=ORIENTED_EDGE('',*,*,#7840,.T.);
#10691=ORIENTED_EDGE('',*,*,#7843,.T.);
#10692=ORIENTED_EDGE('',*,*,#7846,.T.);
#10693=ORIENTED_EDGE('',*,*,#7849,.T.);
#10694=ORIENTED_EDGE('',*,*,#7852,.T.);
#10695=ORIENTED_EDGE('',*,*,#7855,.T.);
#10696=ORIENTED_EDGE('',*,*,#7858,.T.);
#10697=ORIENTED_EDGE('',*,*,#7861,.T.);
#10698=ORIENTED_EDGE('',*,*,#7864,.T.);
#10699=ORIENTED_EDGE('',*,*,#7867,.T.);
#10700=ORIENTED_EDGE('',*,*,#7870,.T.);
#10701=ORIENTED_EDGE('',*,*,#7873,.T.);
#10702=ORIENTED_EDGE('',*,*,#7876,.T.);
#10703=ORIENTED_EDGE('',*,*,#7879,.T.);
#10704=ORIENTED_EDGE('',*,*,#7884,.F.);
#10705=ORIENTED_EDGE('',*,*,#7885,.T.);
#10706=ORIENTED_EDGE('',*,*,#7401,.T.);
#10707=ORIENTED_EDGE('',*,*,#7384,.T.);
#10708=ORIENTED_EDGE('',*,*,#7392,.T.);
#10709=ORIENTED_EDGE('',*,*,#7886,.T.);
#10710=ORIENTED_EDGE('',*,*,#7887,.T.);
#10711=ORIENTED_EDGE('',*,*,#7886,.F.);
#10712=ORIENTED_EDGE('',*,*,#7396,.T.);
#10713=ORIENTED_EDGE('',*,*,#7388,.T.);
#10714=ORIENTED_EDGE('',*,*,#7397,.T.);
#10715=ORIENTED_EDGE('',*,*,#7885,.F.);
#10716=ORIENTED_EDGE('',*,*,#7884,.T.);
#10717=ORIENTED_EDGE('',*,*,#7887,.F.);
#10718=ORIENTED_EDGE('',*,*,#7381,.T.);
#11885=CYLINDRICAL_SURFACE('',#13757,0.425);
#11886=CYLINDRICAL_SURFACE('',#13932,1.);
#12229=ADVANCED_FACE('',(#1620),#11885,.F.);
#12230=ADVANCED_FACE('',(#1621),#1044,.F.);
#12231=ADVANCED_FACE('',(#1622),#1045,.T.);
#12232=ADVANCED_FACE('',(#1623),#1046,.T.);
#12233=ADVANCED_FACE('',(#1624),#1047,.T.);
#12234=ADVANCED_FACE('',(#1625),#1048,.T.);
#12235=ADVANCED_FACE('',(#1626),#1049,.T.);
#12236=ADVANCED_FACE('',(#1627),#1050,.T.);
#12237=ADVANCED_FACE('',(#1628),#1051,.T.);
#12238=ADVANCED_FACE('',(#1629),#1052,.T.);
#12239=ADVANCED_FACE('',(#1630),#1053,.T.);
#12240=ADVANCED_FACE('',(#1631),#1054,.T.);
#12241=ADVANCED_FACE('',(#1632),#1055,.T.);
#12242=ADVANCED_FACE('',(#1633),#1056,.T.);
#12243=ADVANCED_FACE('',(#1634),#1057,.T.);
#12244=ADVANCED_FACE('',(#1635),#1058,.T.);
#12245=ADVANCED_FACE('',(#1636),#1059,.T.);
#12246=ADVANCED_FACE('',(#1637),#1060,.T.);
#12247=ADVANCED_FACE('',(#1638),#1061,.T.);
#12248=ADVANCED_FACE('',(#1639),#1062,.T.);
#12249=ADVANCED_FACE('',(#1640),#1063,.T.);
#12250=ADVANCED_FACE('',(#1641),#1064,.T.);
#12251=ADVANCED_FACE('',(#1642),#1065,.T.);
#12252=ADVANCED_FACE('',(#1643),#1066,.T.);
#12253=ADVANCED_FACE('',(#1644),#1067,.T.);
#12254=ADVANCED_FACE('',(#1645),#1068,.T.);
#12255=ADVANCED_FACE('',(#1646),#1069,.T.);
#12256=ADVANCED_FACE('',(#1647),#1070,.T.);
#12257=ADVANCED_FACE('',(#1648),#1071,.T.);
#12258=ADVANCED_FACE('',(#1649),#1072,.T.);
#12259=ADVANCED_FACE('',(#1650),#1073,.T.);
#12260=ADVANCED_FACE('',(#1651),#1074,.T.);
#12261=ADVANCED_FACE('',(#1652),#1075,.T.);
#12262=ADVANCED_FACE('',(#1653),#1076,.T.);
#12263=ADVANCED_FACE('',(#1654),#1077,.T.);
#12264=ADVANCED_FACE('',(#1655),#1078,.T.);
#12265=ADVANCED_FACE('',(#1656),#1079,.T.);
#12266=ADVANCED_FACE('',(#1657),#1080,.T.);
#12267=ADVANCED_FACE('',(#1658),#1081,.T.);
#12268=ADVANCED_FACE('',(#1659),#1082,.T.);
#12269=ADVANCED_FACE('',(#1660),#1083,.T.);
#12270=ADVANCED_FACE('',(#1661),#1084,.T.);
#12271=ADVANCED_FACE('',(#1662),#1085,.T.);
#12272=ADVANCED_FACE('',(#1663),#1086,.T.);
#12273=ADVANCED_FACE('',(#1664),#1087,.T.);
#12274=ADVANCED_FACE('',(#1665),#1088,.T.);
#12275=ADVANCED_FACE('',(#1666),#1089,.T.);
#12276=ADVANCED_FACE('',(#1667),#1090,.T.);
#12277=ADVANCED_FACE('',(#1668),#1091,.T.);
#12278=ADVANCED_FACE('',(#1669),#1092,.T.);
#12279=ADVANCED_FACE('',(#1670),#1093,.T.);
#12280=ADVANCED_FACE('',(#1671),#1094,.T.);
#12281=ADVANCED_FACE('',(#1672),#1095,.T.);
#12282=ADVANCED_FACE('',(#1673),#1096,.T.);
#12283=ADVANCED_FACE('',(#1674),#1097,.T.);
#12284=ADVANCED_FACE('',(#1675),#1098,.T.);
#12285=ADVANCED_FACE('',(#1676),#1099,.T.);
#12286=ADVANCED_FACE('',(#1677),#1100,.T.);
#12287=ADVANCED_FACE('',(#1678),#1101,.T.);
#12288=ADVANCED_FACE('',(#1679),#1102,.T.);
#12289=ADVANCED_FACE('',(#1680),#1103,.T.);
#12290=ADVANCED_FACE('',(#1681),#1104,.T.);
#12291=ADVANCED_FACE('',(#1682),#1105,.T.);
#12292=ADVANCED_FACE('',(#1683),#1106,.T.);
#12293=ADVANCED_FACE('',(#1684),#1107,.T.);
#12294=ADVANCED_FACE('',(#1685),#1108,.T.);
#12295=ADVANCED_FACE('',(#1686),#1109,.T.);
#12296=ADVANCED_FACE('',(#1687),#1110,.T.);
#12297=ADVANCED_FACE('',(#1688),#1111,.T.);
#12298=ADVANCED_FACE('',(#1689),#1112,.T.);
#12299=ADVANCED_FACE('',(#1690),#1113,.T.);
#12300=ADVANCED_FACE('',(#1691),#1114,.T.);
#12301=ADVANCED_FACE('',(#1692),#1115,.T.);
#12302=ADVANCED_FACE('',(#1693),#1116,.T.);
#12303=ADVANCED_FACE('',(#1694),#1117,.T.);
#12304=ADVANCED_FACE('',(#1695),#1118,.T.);
#12305=ADVANCED_FACE('',(#1696),#1119,.T.);
#12306=ADVANCED_FACE('',(#1697),#1120,.T.);
#12307=ADVANCED_FACE('',(#1698),#1121,.T.);
#12308=ADVANCED_FACE('',(#1699),#1122,.T.);
#12309=ADVANCED_FACE('',(#1700),#1123,.T.);
#12310=ADVANCED_FACE('',(#1701),#1124,.T.);
#12311=ADVANCED_FACE('',(#1702),#1125,.T.);
#12312=ADVANCED_FACE('',(#1703),#1126,.T.);
#12313=ADVANCED_FACE('',(#1704),#1127,.T.);
#12314=ADVANCED_FACE('',(#1705),#1128,.T.);
#12315=ADVANCED_FACE('',(#1706),#1129,.T.);
#12316=ADVANCED_FACE('',(#1707),#1130,.T.);
#12317=ADVANCED_FACE('',(#1708),#1131,.T.);
#12318=ADVANCED_FACE('',(#1709),#1132,.T.);
#12319=ADVANCED_FACE('',(#1710),#1133,.T.);
#12320=ADVANCED_FACE('',(#1711),#1134,.T.);
#12321=ADVANCED_FACE('',(#1712),#1135,.T.);
#12322=ADVANCED_FACE('',(#1713),#1136,.T.);
#12323=ADVANCED_FACE('',(#1714),#1137,.T.);
#12324=ADVANCED_FACE('',(#1715),#1138,.T.);
#12325=ADVANCED_FACE('',(#1716),#1139,.T.);
#12326=ADVANCED_FACE('',(#1717),#1140,.T.);
#12327=ADVANCED_FACE('',(#1718),#1141,.T.);
#12328=ADVANCED_FACE('',(#1719),#1142,.T.);
#12329=ADVANCED_FACE('',(#1720),#1143,.T.);
#12330=ADVANCED_FACE('',(#1721),#1144,.T.);
#12331=ADVANCED_FACE('',(#1722),#1145,.T.);
#12332=ADVANCED_FACE('',(#1723),#1146,.T.);
#12333=ADVANCED_FACE('',(#1724),#1147,.T.);
#12334=ADVANCED_FACE('',(#1725),#1148,.T.);
#12335=ADVANCED_FACE('',(#1726),#1149,.T.);
#12336=ADVANCED_FACE('',(#1727),#1150,.T.);
#12337=ADVANCED_FACE('',(#1728),#1151,.T.);
#12338=ADVANCED_FACE('',(#1729),#1152,.T.);
#12339=ADVANCED_FACE('',(#1730),#1153,.T.);
#12340=ADVANCED_FACE('',(#1731),#1154,.T.);
#12341=ADVANCED_FACE('',(#1732),#1155,.T.);
#12342=ADVANCED_FACE('',(#1733),#1156,.T.);
#12343=ADVANCED_FACE('',(#1734),#1157,.T.);
#12344=ADVANCED_FACE('',(#1735),#1158,.T.);
#12345=ADVANCED_FACE('',(#1736),#1159,.T.);
#12346=ADVANCED_FACE('',(#1737),#1160,.T.);
#12347=ADVANCED_FACE('',(#1738),#1161,.T.);
#12348=ADVANCED_FACE('',(#1739),#1162,.T.);
#12349=ADVANCED_FACE('',(#1740),#1163,.T.);
#12350=ADVANCED_FACE('',(#1741),#1164,.T.);
#12351=ADVANCED_FACE('',(#1742),#1165,.T.);
#12352=ADVANCED_FACE('',(#1743),#1166,.T.);
#12353=ADVANCED_FACE('',(#1744),#1167,.T.);
#12354=ADVANCED_FACE('',(#1745),#1168,.T.);
#12355=ADVANCED_FACE('',(#1746),#1169,.T.);
#12356=ADVANCED_FACE('',(#1747),#1170,.T.);
#12357=ADVANCED_FACE('',(#1748),#1171,.T.);
#12358=ADVANCED_FACE('',(#1749),#1172,.T.);
#12359=ADVANCED_FACE('',(#1750),#1173,.T.);
#12360=ADVANCED_FACE('',(#1751),#1174,.T.);
#12361=ADVANCED_FACE('',(#1752),#1175,.T.);
#12362=ADVANCED_FACE('',(#1753),#1176,.T.);
#12363=ADVANCED_FACE('',(#1754),#1177,.T.);
#12364=ADVANCED_FACE('',(#1755),#1178,.T.);
#12365=ADVANCED_FACE('',(#1756),#1179,.T.);
#12366=ADVANCED_FACE('',(#1757),#1180,.T.);
#12367=ADVANCED_FACE('',(#1758),#1181,.T.);
#12368=ADVANCED_FACE('',(#1759),#1182,.T.);
#12369=ADVANCED_FACE('',(#1760),#1183,.T.);
#12370=ADVANCED_FACE('',(#1761),#1184,.T.);
#12371=ADVANCED_FACE('',(#1762),#1185,.T.);
#12372=ADVANCED_FACE('',(#1763),#1186,.T.);
#12373=ADVANCED_FACE('',(#1764),#1187,.T.);
#12374=ADVANCED_FACE('',(#1765),#1188,.T.);
#12375=ADVANCED_FACE('',(#1766),#1189,.T.);
#12376=ADVANCED_FACE('',(#1767),#1190,.T.);
#12377=ADVANCED_FACE('',(#1768),#1191,.T.);
#12378=ADVANCED_FACE('',(#1769),#1192,.T.);
#12379=ADVANCED_FACE('',(#1770),#1193,.T.);
#12380=ADVANCED_FACE('',(#1771),#1194,.T.);
#12381=ADVANCED_FACE('',(#1772),#1195,.T.);
#12382=ADVANCED_FACE('',(#1773),#1196,.T.);
#12383=ADVANCED_FACE('',(#1774),#1197,.T.);
#12384=ADVANCED_FACE('',(#1775),#1198,.T.);
#12385=ADVANCED_FACE('',(#1776),#1199,.T.);
#12386=ADVANCED_FACE('',(#1777),#1200,.T.);
#12387=ADVANCED_FACE('',(#1778),#1201,.T.);
#12388=ADVANCED_FACE('',(#1779),#1202,.T.);
#12389=ADVANCED_FACE('',(#1780),#1203,.T.);
#12390=ADVANCED_FACE('',(#1781),#1204,.T.);
#12391=ADVANCED_FACE('',(#1782),#1205,.T.);
#12392=ADVANCED_FACE('',(#1783),#1206,.T.);
#12393=ADVANCED_FACE('',(#1784),#1207,.T.);
#12394=ADVANCED_FACE('',(#1785),#1208,.T.);
#12395=ADVANCED_FACE('',(#1786),#1209,.T.);
#12396=ADVANCED_FACE('',(#1787),#1210,.T.);
#12397=ADVANCED_FACE('',(#1788),#1211,.F.);
#12398=ADVANCED_FACE('',(#1789),#11886,.T.);
#12399=ADVANCED_FACE('',(#1790),#1212,.T.);
#12400=ADVANCED_FACE('',(#1791,#846),#1213,.F.);
#12668=CLOSED_SHELL('',(#12229,#12230,#12231,#12232,#12233,#12234,#12235,
#12236,#12237,#12238,#12239,#12240,#12241,#12242,#12243,#12244,#12245,#12246,
#12247,#12248,#12249,#12250,#12251,#12252,#12253,#12254,#12255,#12256,#12257,
#12258,#12259,#12260,#12261,#12262,#12263,#12264,#12265,#12266,#12267,#12268,
#12269,#12270,#12271,#12272,#12273,#12274,#12275,#12276,#12277,#12278,#12279,
#12280,#12281,#12282,#12283,#12284,#12285,#12286,#12287,#12288,#12289,#12290,
#12291,#12292,#12293,#12294,#12295,#12296,#12297,#12298,#12299,#12300,#12301,
#12302,#12303,#12304,#12305,#12306,#12307,#12308,#12309,#12310,#12311,#12312,
#12313,#12314,#12315,#12316,#12317,#12318,#12319,#12320,#12321,#12322,#12323,
#12324,#12325,#12326,#12327,#12328,#12329,#12330,#12331,#12332,#12333,#12334,
#12335,#12336,#12337,#12338,#12339,#12340,#12341,#12342,#12343,#12344,#12345,
#12346,#12347,#12348,#12349,#12350,#12351,#12352,#12353,#12354,#12355,#12356,
#12357,#12358,#12359,#12360,#12361,#12362,#12363,#12364,#12365,#12366,#12367,
#12368,#12369,#12370,#12371,#12372,#12373,#12374,#12375,#12376,#12377,#12378,
#12379,#12380,#12381,#12382,#12383,#12384,#12385,#12386,#12387,#12388,#12389,
#12390,#12391,#12392,#12393,#12394,#12395,#12396,#12397,#12398,#12399,#12400));
#13756=AXIS2_PLACEMENT_3D('',#19757,#15861,#15862);
#13757=AXIS2_PLACEMENT_3D('',#19758,#15863,#15864);
#13758=AXIS2_PLACEMENT_3D('',#19760,#15865,#15866);
#13759=AXIS2_PLACEMENT_3D('',#19763,#15868,#15869);
#13760=AXIS2_PLACEMENT_3D('',#19764,#15870,#15871);
#13761=AXIS2_PLACEMENT_3D('',#19765,#15872,#15873);
#13762=AXIS2_PLACEMENT_3D('',#19774,#15878,#15879);
#13763=AXIS2_PLACEMENT_3D('',#19783,#15884,#15885);
#13764=AXIS2_PLACEMENT_3D('',#19785,#15886,#15887);
#13765=AXIS2_PLACEMENT_3D('',#19791,#15891,#15892);
#13766=AXIS2_PLACEMENT_3D('',#19792,#15893,#15894);
#13767=AXIS2_PLACEMENT_3D('',#19794,#15895,#15896);
#13768=AXIS2_PLACEMENT_3D('',#19800,#15900,#15901);
#13769=AXIS2_PLACEMENT_3D('',#19801,#15902,#15903);
#13770=AXIS2_PLACEMENT_3D('',#19807,#15907,#15908);
#13771=AXIS2_PLACEMENT_3D('',#19813,#15912,#15913);
#13772=AXIS2_PLACEMENT_3D('',#19819,#15917,#15918);
#13773=AXIS2_PLACEMENT_3D('',#19825,#15922,#15923);
#13774=AXIS2_PLACEMENT_3D('',#19831,#15927,#15928);
#13775=AXIS2_PLACEMENT_3D('',#19837,#15932,#15933);
#13776=AXIS2_PLACEMENT_3D('',#19843,#15937,#15938);
#13777=AXIS2_PLACEMENT_3D('',#19849,#15942,#15943);
#13778=AXIS2_PLACEMENT_3D('',#19855,#15947,#15948);
#13779=AXIS2_PLACEMENT_3D('',#19861,#15952,#15953);
#13780=AXIS2_PLACEMENT_3D('',#19867,#15957,#15958);
#13781=AXIS2_PLACEMENT_3D('',#19873,#15962,#15963);
#13782=AXIS2_PLACEMENT_3D('',#19879,#15967,#15968);
#13783=AXIS2_PLACEMENT_3D('',#19885,#15972,#15973);
#13784=AXIS2_PLACEMENT_3D('',#19891,#15977,#15978);
#13785=AXIS2_PLACEMENT_3D('',#19897,#15982,#15983);
#13786=AXIS2_PLACEMENT_3D('',#19903,#15987,#15988);
#13787=AXIS2_PLACEMENT_3D('',#19909,#15992,#15993);
#13788=AXIS2_PLACEMENT_3D('',#19915,#15997,#15998);
#13789=AXIS2_PLACEMENT_3D('',#19921,#16002,#16003);
#13790=AXIS2_PLACEMENT_3D('',#19927,#16007,#16008);
#13791=AXIS2_PLACEMENT_3D('',#19933,#16012,#16013);
#13792=AXIS2_PLACEMENT_3D('',#19939,#16017,#16018);
#13793=AXIS2_PLACEMENT_3D('',#19945,#16022,#16023);
#13794=AXIS2_PLACEMENT_3D('',#19951,#16027,#16028);
#13795=AXIS2_PLACEMENT_3D('',#19957,#16032,#16033);
#13796=AXIS2_PLACEMENT_3D('',#19963,#16037,#16038);
#13797=AXIS2_PLACEMENT_3D('',#19969,#16042,#16043);
#13798=AXIS2_PLACEMENT_3D('',#19975,#16047,#16048);
#13799=AXIS2_PLACEMENT_3D('',#19981,#16052,#16053);
#13800=AXIS2_PLACEMENT_3D('',#19987,#16057,#16058);
#13801=AXIS2_PLACEMENT_3D('',#19993,#16062,#16063);
#13802=AXIS2_PLACEMENT_3D('',#19999,#16067,#16068);
#13803=AXIS2_PLACEMENT_3D('',#20005,#16072,#16073);
#13804=AXIS2_PLACEMENT_3D('',#20011,#16077,#16078);
#13805=AXIS2_PLACEMENT_3D('',#20017,#16082,#16083);
#13806=AXIS2_PLACEMENT_3D('',#20023,#16087,#16088);
#13807=AXIS2_PLACEMENT_3D('',#20029,#16092,#16093);
#13808=AXIS2_PLACEMENT_3D('',#20035,#16097,#16098);
#13809=AXIS2_PLACEMENT_3D('',#20041,#16102,#16103);
#13810=AXIS2_PLACEMENT_3D('',#20047,#16107,#16108);
#13811=AXIS2_PLACEMENT_3D('',#20053,#16112,#16113);
#13812=AXIS2_PLACEMENT_3D('',#20059,#16117,#16118);
#13813=AXIS2_PLACEMENT_3D('',#20065,#16122,#16123);
#13814=AXIS2_PLACEMENT_3D('',#20071,#16127,#16128);
#13815=AXIS2_PLACEMENT_3D('',#20077,#16132,#16133);
#13816=AXIS2_PLACEMENT_3D('',#20083,#16137,#16138);
#13817=AXIS2_PLACEMENT_3D('',#20089,#16142,#16143);
#13818=AXIS2_PLACEMENT_3D('',#20095,#16147,#16148);
#13819=AXIS2_PLACEMENT_3D('',#20101,#16152,#16153);
#13820=AXIS2_PLACEMENT_3D('',#20107,#16157,#16158);
#13821=AXIS2_PLACEMENT_3D('',#20113,#16162,#16163);
#13822=AXIS2_PLACEMENT_3D('',#20119,#16167,#16168);
#13823=AXIS2_PLACEMENT_3D('',#20125,#16172,#16173);
#13824=AXIS2_PLACEMENT_3D('',#20131,#16177,#16178);
#13825=AXIS2_PLACEMENT_3D('',#20137,#16182,#16183);
#13826=AXIS2_PLACEMENT_3D('',#20143,#16187,#16188);
#13827=AXIS2_PLACEMENT_3D('',#20149,#16192,#16193);
#13828=AXIS2_PLACEMENT_3D('',#20155,#16197,#16198);
#13829=AXIS2_PLACEMENT_3D('',#20161,#16202,#16203);
#13830=AXIS2_PLACEMENT_3D('',#20167,#16207,#16208);
#13831=AXIS2_PLACEMENT_3D('',#20173,#16212,#16213);
#13832=AXIS2_PLACEMENT_3D('',#20179,#16217,#16218);
#13833=AXIS2_PLACEMENT_3D('',#20185,#16222,#16223);
#13834=AXIS2_PLACEMENT_3D('',#20191,#16227,#16228);
#13835=AXIS2_PLACEMENT_3D('',#20197,#16232,#16233);
#13836=AXIS2_PLACEMENT_3D('',#20203,#16237,#16238);
#13837=AXIS2_PLACEMENT_3D('',#20209,#16242,#16243);
#13838=AXIS2_PLACEMENT_3D('',#20215,#16247,#16248);
#13839=AXIS2_PLACEMENT_3D('',#20221,#16252,#16253);
#13840=AXIS2_PLACEMENT_3D('',#20227,#16257,#16258);
#13841=AXIS2_PLACEMENT_3D('',#20233,#16262,#16263);
#13842=AXIS2_PLACEMENT_3D('',#20239,#16267,#16268);
#13843=AXIS2_PLACEMENT_3D('',#20245,#16272,#16273);
#13844=AXIS2_PLACEMENT_3D('',#20251,#16277,#16278);
#13845=AXIS2_PLACEMENT_3D('',#20257,#16282,#16283);
#13846=AXIS2_PLACEMENT_3D('',#20263,#16287,#16288);
#13847=AXIS2_PLACEMENT_3D('',#20269,#16292,#16293);
#13848=AXIS2_PLACEMENT_3D('',#20275,#16297,#16298);
#13849=AXIS2_PLACEMENT_3D('',#20281,#16302,#16303);
#13850=AXIS2_PLACEMENT_3D('',#20287,#16307,#16308);
#13851=AXIS2_PLACEMENT_3D('',#20293,#16312,#16313);
#13852=AXIS2_PLACEMENT_3D('',#20299,#16317,#16318);
#13853=AXIS2_PLACEMENT_3D('',#20305,#16322,#16323);
#13854=AXIS2_PLACEMENT_3D('',#20311,#16327,#16328);
#13855=AXIS2_PLACEMENT_3D('',#20317,#16332,#16333);
#13856=AXIS2_PLACEMENT_3D('',#20323,#16337,#16338);
#13857=AXIS2_PLACEMENT_3D('',#20329,#16342,#16343);
#13858=AXIS2_PLACEMENT_3D('',#20335,#16347,#16348);
#13859=AXIS2_PLACEMENT_3D('',#20341,#16352,#16353);
#13860=AXIS2_PLACEMENT_3D('',#20347,#16357,#16358);
#13861=AXIS2_PLACEMENT_3D('',#20353,#16362,#16363);
#13862=AXIS2_PLACEMENT_3D('',#20359,#16367,#16368);
#13863=AXIS2_PLACEMENT_3D('',#20365,#16372,#16373);
#13864=AXIS2_PLACEMENT_3D('',#20371,#16377,#16378);
#13865=AXIS2_PLACEMENT_3D('',#20377,#16382,#16383);
#13866=AXIS2_PLACEMENT_3D('',#20383,#16387,#16388);
#13867=AXIS2_PLACEMENT_3D('',#20389,#16392,#16393);
#13868=AXIS2_PLACEMENT_3D('',#20395,#16397,#16398);
#13869=AXIS2_PLACEMENT_3D('',#20401,#16402,#16403);
#13870=AXIS2_PLACEMENT_3D('',#20407,#16407,#16408);
#13871=AXIS2_PLACEMENT_3D('',#20413,#16412,#16413);
#13872=AXIS2_PLACEMENT_3D('',#20419,#16417,#16418);
#13873=AXIS2_PLACEMENT_3D('',#20425,#16422,#16423);
#13874=AXIS2_PLACEMENT_3D('',#20431,#16427,#16428);
#13875=AXIS2_PLACEMENT_3D('',#20437,#16432,#16433);
#13876=AXIS2_PLACEMENT_3D('',#20443,#16437,#16438);
#13877=AXIS2_PLACEMENT_3D('',#20449,#16442,#16443);
#13878=AXIS2_PLACEMENT_3D('',#20455,#16447,#16448);
#13879=AXIS2_PLACEMENT_3D('',#20461,#16452,#16453);
#13880=AXIS2_PLACEMENT_3D('',#20467,#16457,#16458);
#13881=AXIS2_PLACEMENT_3D('',#20473,#16462,#16463);
#13882=AXIS2_PLACEMENT_3D('',#20479,#16467,#16468);
#13883=AXIS2_PLACEMENT_3D('',#20485,#16472,#16473);
#13884=AXIS2_PLACEMENT_3D('',#20491,#16477,#16478);
#13885=AXIS2_PLACEMENT_3D('',#20497,#16482,#16483);
#13886=AXIS2_PLACEMENT_3D('',#20503,#16487,#16488);
#13887=AXIS2_PLACEMENT_3D('',#20509,#16492,#16493);
#13888=AXIS2_PLACEMENT_3D('',#20515,#16497,#16498);
#13889=AXIS2_PLACEMENT_3D('',#20521,#16502,#16503);
#13890=AXIS2_PLACEMENT_3D('',#20527,#16507,#16508);
#13891=AXIS2_PLACEMENT_3D('',#20533,#16512,#16513);
#13892=AXIS2_PLACEMENT_3D('',#20539,#16517,#16518);
#13893=AXIS2_PLACEMENT_3D('',#20545,#16522,#16523);
#13894=AXIS2_PLACEMENT_3D('',#20551,#16527,#16528);
#13895=AXIS2_PLACEMENT_3D('',#20557,#16532,#16533);
#13896=AXIS2_PLACEMENT_3D('',#20563,#16537,#16538);
#13897=AXIS2_PLACEMENT_3D('',#20569,#16542,#16543);
#13898=AXIS2_PLACEMENT_3D('',#20575,#16547,#16548);
#13899=AXIS2_PLACEMENT_3D('',#20581,#16552,#16553);
#13900=AXIS2_PLACEMENT_3D('',#20587,#16557,#16558);
#13901=AXIS2_PLACEMENT_3D('',#20593,#16562,#16563);
#13902=AXIS2_PLACEMENT_3D('',#20599,#16567,#16568);
#13903=AXIS2_PLACEMENT_3D('',#20605,#16572,#16573);
#13904=AXIS2_PLACEMENT_3D('',#20611,#16577,#16578);
#13905=AXIS2_PLACEMENT_3D('',#20617,#16582,#16583);
#13906=AXIS2_PLACEMENT_3D('',#20623,#16587,#16588);
#13907=AXIS2_PLACEMENT_3D('',#20629,#16592,#16593);
#13908=AXIS2_PLACEMENT_3D('',#20635,#16597,#16598);
#13909=AXIS2_PLACEMENT_3D('',#20641,#16602,#16603);
#13910=AXIS2_PLACEMENT_3D('',#20647,#16607,#16608);
#13911=AXIS2_PLACEMENT_3D('',#20653,#16612,#16613);
#13912=AXIS2_PLACEMENT_3D('',#20659,#16617,#16618);
#13913=AXIS2_PLACEMENT_3D('',#20665,#16622,#16623);
#13914=AXIS2_PLACEMENT_3D('',#20671,#16627,#16628);
#13915=AXIS2_PLACEMENT_3D('',#20677,#16632,#16633);
#13916=AXIS2_PLACEMENT_3D('',#20683,#16637,#16638);
#13917=AXIS2_PLACEMENT_3D('',#20689,#16642,#16643);
#13918=AXIS2_PLACEMENT_3D('',#20695,#16647,#16648);
#13919=AXIS2_PLACEMENT_3D('',#20701,#16652,#16653);
#13920=AXIS2_PLACEMENT_3D('',#20707,#16657,#16658);
#13921=AXIS2_PLACEMENT_3D('',#20713,#16662,#16663);
#13922=AXIS2_PLACEMENT_3D('',#20719,#16667,#16668);
#13923=AXIS2_PLACEMENT_3D('',#20725,#16672,#16673);
#13924=AXIS2_PLACEMENT_3D('',#20731,#16677,#16678);
#13925=AXIS2_PLACEMENT_3D('',#20737,#16682,#16683);
#13926=AXIS2_PLACEMENT_3D('',#20743,#16687,#16688);
#13927=AXIS2_PLACEMENT_3D('',#20749,#16692,#16693);
#13928=AXIS2_PLACEMENT_3D('',#20755,#16697,#16698);
#13929=AXIS2_PLACEMENT_3D('',#20761,#16702,#16703);
#13930=AXIS2_PLACEMENT_3D('',#20764,#16706,#16707);
#13931=AXIS2_PLACEMENT_3D('',#20765,#16708,#16709);
#13932=AXIS2_PLACEMENT_3D('',#20766,#16710,#16711);
#13933=AXIS2_PLACEMENT_3D('',#20768,#16712,#16713);
#13934=AXIS2_PLACEMENT_3D('',#20772,#16716,#16717);
#13935=AXIS2_PLACEMENT_3D('',#20773,#16718,#16719);
#13936=AXIS2_PLACEMENT_3D('',#20774,#16720,#16721);
#15861=DIRECTION('axis',(0.,0.,1.));
#15862=DIRECTION('refdir',(1.,0.,0.));
#15863=DIRECTION('center_axis',(0.,0.,1.));
#15864=DIRECTION('ref_axis',(1.,0.,0.));
#15865=DIRECTION('center_axis',(0.,0.,1.));
#15866=DIRECTION('ref_axis',(1.,0.,0.));
#15867=DIRECTION('',(0.,0.,1.));
#15868=DIRECTION('center_axis',(0.,0.,1.));
#15869=DIRECTION('ref_axis',(1.,0.,0.));
#15870=DIRECTION('center_axis',(0.,0.,1.));
#15871=DIRECTION('ref_axis',(1.,0.,0.));
#15872=DIRECTION('center_axis',(1.,0.,0.));
#15873=DIRECTION('ref_axis',(0.,0.,-1.));
#15874=DIRECTION('',(0.,0.,-1.));
#15875=DIRECTION('',(0.,1.,0.));
#15876=DIRECTION('',(0.,0.,1.));
#15877=DIRECTION('',(0.,1.,0.));
#15878=DIRECTION('center_axis',(1.,0.,0.));
#15879=DIRECTION('ref_axis',(0.,0.,-1.));
#15880=DIRECTION('',(0.,0.,1.));
#15881=DIRECTION('',(0.,1.,0.));
#15882=DIRECTION('',(0.,0.,-1.));
#15883=DIRECTION('',(0.,1.,0.));
#15884=DIRECTION('center_axis',(0.,0.,-1.));
#15885=DIRECTION('ref_axis',(-1.,0.,0.));
#15886=DIRECTION('center_axis',(0.,0.,-1.));
#15887=DIRECTION('ref_axis',(1.,0.,0.));
#15888=DIRECTION('',(1.,0.,0.));
#15889=DIRECTION('',(0.,1.,0.));
#15890=DIRECTION('',(-1.,0.,0.));
#15891=DIRECTION('center_axis',(0.,0.,-1.));
#15892=DIRECTION('ref_axis',(1.,0.,0.));
#15893=DIRECTION('center_axis',(0.,0.,1.));
#15894=DIRECTION('ref_axis',(1.,0.,0.));
#15895=DIRECTION('center_axis',(0.,0.,1.));
#15896=DIRECTION('ref_axis',(1.,0.,0.));
#15897=DIRECTION('',(1.,0.,0.));
#15898=DIRECTION('',(0.,1.,0.));
#15899=DIRECTION('',(-1.,0.,0.));
#15900=DIRECTION('center_axis',(0.,0.,1.));
#15901=DIRECTION('ref_axis',(1.,0.,0.));
#15902=DIRECTION('center_axis',(-1.,0.,0.));
#15903=DIRECTION('ref_axis',(0.,0.,1.));
#15904=DIRECTION('',(0.,0.,-1.));
#15905=DIRECTION('',(0.,0.,1.));
#15906=DIRECTION('',(0.,1.,0.));
#15907=DIRECTION('center_axis',(-0.342020143325675,0.,0.939692620785906));
#15908=DIRECTION('ref_axis',(0.939692620785906,0.,0.342020143325675));
#15909=DIRECTION('',(-0.939692620785906,0.,-0.342020143325675));
#15910=DIRECTION('',(0.939692620785906,0.,0.342020143325675));
#15911=DIRECTION('',(0.,1.,0.));
#15912=DIRECTION('center_axis',(-1.,0.,0.));
#15913=DIRECTION('ref_axis',(0.,0.,1.));
#15914=DIRECTION('',(0.,0.,-1.));
#15915=DIRECTION('',(0.,0.,1.));
#15916=DIRECTION('',(0.,1.,0.));
#15917=DIRECTION('center_axis',(-0.342020143325675,0.,-0.939692620785906));
#15918=DIRECTION('ref_axis',(-0.939692620785906,0.,0.342020143325675));
#15919=DIRECTION('',(0.939692620785906,0.,-0.342020143325675));
#15920=DIRECTION('',(-0.939692620785906,0.,0.342020143325675));
#15921=DIRECTION('',(0.,1.,0.));
#15922=DIRECTION('center_axis',(-1.,0.,0.));
#15923=DIRECTION('ref_axis',(0.,0.,1.));
#15924=DIRECTION('',(0.,0.,-1.));
#15925=DIRECTION('',(0.,0.,1.));
#15926=DIRECTION('',(0.,1.,0.));
#15927=DIRECTION('center_axis',(-0.342020143325675,0.,0.939692620785906));
#15928=DIRECTION('ref_axis',(0.939692620785906,0.,0.342020143325675));
#15929=DIRECTION('',(-0.939692620785906,0.,-0.342020143325675));
#15930=DIRECTION('',(0.939692620785906,0.,0.342020143325675));
#15931=DIRECTION('',(0.,1.,0.));
#15932=DIRECTION('center_axis',(-1.,0.,0.));
#15933=DIRECTION('ref_axis',(0.,0.,1.));
#15934=DIRECTION('',(0.,0.,-1.));
#15935=DIRECTION('',(0.,0.,1.));
#15936=DIRECTION('',(0.,1.,0.));
#15937=DIRECTION('center_axis',(-0.342020143325675,0.,-0.939692620785906));
#15938=DIRECTION('ref_axis',(-0.939692620785906,0.,0.342020143325675));
#15939=DIRECTION('',(0.939692620785906,0.,-0.342020143325675));
#15940=DIRECTION('',(-0.939692620785906,0.,0.342020143325675));
#15941=DIRECTION('',(0.,1.,0.));
#15942=DIRECTION('center_axis',(-1.,0.,0.));
#15943=DIRECTION('ref_axis',(0.,0.,1.));
#15944=DIRECTION('',(0.,0.,-1.));
#15945=DIRECTION('',(0.,0.,1.));
#15946=DIRECTION('',(0.,1.,0.));
#15947=DIRECTION('center_axis',(-0.342020143325675,0.,0.939692620785906));
#15948=DIRECTION('ref_axis',(0.939692620785906,0.,0.342020143325675));
#15949=DIRECTION('',(-0.939692620785906,0.,-0.342020143325675));
#15950=DIRECTION('',(0.939692620785906,0.,0.342020143325675));
#15951=DIRECTION('',(0.,1.,0.));
#15952=DIRECTION('center_axis',(-1.,0.,0.));
#15953=DIRECTION('ref_axis',(0.,0.,1.));
#15954=DIRECTION('',(0.,0.,-1.));
#15955=DIRECTION('',(0.,0.,1.));
#15956=DIRECTION('',(0.,1.,0.));
#15957=DIRECTION('center_axis',(-0.342020143325675,0.,-0.939692620785906));
#15958=DIRECTION('ref_axis',(-0.939692620785906,0.,0.342020143325675));
#15959=DIRECTION('',(0.939692620785906,0.,-0.342020143325675));
#15960=DIRECTION('',(-0.939692620785906,0.,0.342020143325675));
#15961=DIRECTION('',(0.,1.,0.));
#15962=DIRECTION('center_axis',(-1.,0.,0.));
#15963=DIRECTION('ref_axis',(0.,0.,1.));
#15964=DIRECTION('',(0.,0.,-1.));
#15965=DIRECTION('',(0.,0.,1.));
#15966=DIRECTION('',(0.,1.,0.));
#15967=DIRECTION('center_axis',(-0.342020143325675,0.,0.939692620785906));
#15968=DIRECTION('ref_axis',(0.939692620785906,0.,0.342020143325675));
#15969=DIRECTION('',(-0.939692620785906,0.,-0.342020143325675));
#15970=DIRECTION('',(0.939692620785906,0.,0.342020143325675));
#15971=DIRECTION('',(0.,1.,0.));
#15972=DIRECTION('center_axis',(-1.,0.,0.));
#15973=DIRECTION('ref_axis',(0.,0.,1.));
#15974=DIRECTION('',(0.,0.,-1.));
#15975=DIRECTION('',(0.,0.,1.));
#15976=DIRECTION('',(0.,1.,0.));
#15977=DIRECTION('center_axis',(-0.342020143325675,0.,-0.939692620785906));
#15978=DIRECTION('ref_axis',(-0.939692620785906,0.,0.342020143325675));
#15979=DIRECTION('',(0.939692620785906,0.,-0.342020143325675));
#15980=DIRECTION('',(-0.939692620785906,0.,0.342020143325675));
#15981=DIRECTION('',(0.,1.,0.));
#15982=DIRECTION('center_axis',(-1.,0.,0.));
#15983=DIRECTION('ref_axis',(0.,0.,1.));
#15984=DIRECTION('',(0.,0.,-1.));
#15985=DIRECTION('',(0.,0.,1.));
#15986=DIRECTION('',(0.,1.,0.));
#15987=DIRECTION('center_axis',(-0.342020143325662,0.,0.939692620785911));
#15988=DIRECTION('ref_axis',(0.939692620785911,0.,0.342020143325662));
#15989=DIRECTION('',(-0.939692620785911,0.,-0.342020143325662));
#15990=DIRECTION('',(0.939692620785911,0.,0.342020143325662));
#15991=DIRECTION('',(0.,1.,0.));
#15992=DIRECTION('center_axis',(-1.,0.,0.));
#15993=DIRECTION('ref_axis',(0.,0.,1.));
#15994=DIRECTION('',(0.,0.,-1.));
#15995=DIRECTION('',(0.,0.,1.));
#15996=DIRECTION('',(0.,1.,0.));
#15997=DIRECTION('center_axis',(-0.342020143325662,0.,-0.939692620785911));
#15998=DIRECTION('ref_axis',(-0.939692620785911,0.,0.342020143325662));
#15999=DIRECTION('',(0.939692620785911,0.,-0.342020143325662));
#16000=DIRECTION('',(-0.939692620785911,0.,0.342020143325662));
#16001=DIRECTION('',(0.,1.,0.));
#16002=DIRECTION('center_axis',(-1.,0.,0.));
#16003=DIRECTION('ref_axis',(0.,0.,1.));
#16004=DIRECTION('',(0.,0.,-1.));
#16005=DIRECTION('',(0.,0.,1.));
#16006=DIRECTION('',(0.,1.,0.));
#16007=DIRECTION('center_axis',(-0.342020143325662,0.,0.939692620785911));
#16008=DIRECTION('ref_axis',(0.939692620785911,0.,0.342020143325662));
#16009=DIRECTION('',(-0.939692620785911,0.,-0.342020143325662));
#16010=DIRECTION('',(0.939692620785911,0.,0.342020143325662));
#16011=DIRECTION('',(0.,1.,0.));
#16012=DIRECTION('center_axis',(-1.,0.,0.));
#16013=DIRECTION('ref_axis',(0.,0.,1.));
#16014=DIRECTION('',(0.,0.,-1.));
#16015=DIRECTION('',(0.,0.,1.));
#16016=DIRECTION('',(0.,1.,0.));
#16017=DIRECTION('center_axis',(-0.342020143325662,0.,-0.939692620785911));
#16018=DIRECTION('ref_axis',(-0.939692620785911,0.,0.342020143325662));
#16019=DIRECTION('',(0.939692620785911,0.,-0.342020143325662));
#16020=DIRECTION('',(-0.939692620785911,0.,0.342020143325662));
#16021=DIRECTION('',(0.,1.,0.));
#16022=DIRECTION('center_axis',(-1.,0.,0.));
#16023=DIRECTION('ref_axis',(0.,0.,1.));
#16024=DIRECTION('',(0.,0.,-1.));
#16025=DIRECTION('',(0.,0.,1.));
#16026=DIRECTION('',(0.,1.,0.));
#16027=DIRECTION('center_axis',(-0.342020143325662,0.,0.939692620785911));
#16028=DIRECTION('ref_axis',(0.939692620785911,0.,0.342020143325662));
#16029=DIRECTION('',(-0.939692620785911,0.,-0.342020143325662));
#16030=DIRECTION('',(0.939692620785911,0.,0.342020143325662));
#16031=DIRECTION('',(0.,1.,0.));
#16032=DIRECTION('center_axis',(-1.,0.,0.));
#16033=DIRECTION('ref_axis',(0.,0.,1.));
#16034=DIRECTION('',(0.,0.,-1.));
#16035=DIRECTION('',(0.,0.,1.));
#16036=DIRECTION('',(0.,1.,0.));
#16037=DIRECTION('center_axis',(-0.342020143325662,0.,-0.939692620785911));
#16038=DIRECTION('ref_axis',(-0.939692620785911,0.,0.342020143325662));
#16039=DIRECTION('',(0.939692620785911,0.,-0.342020143325662));
#16040=DIRECTION('',(-0.939692620785911,0.,0.342020143325662));
#16041=DIRECTION('',(0.,1.,0.));
#16042=DIRECTION('center_axis',(-1.,0.,0.));
#16043=DIRECTION('ref_axis',(0.,0.,1.));
#16044=DIRECTION('',(0.,0.,-1.));
#16045=DIRECTION('',(0.,0.,1.));
#16046=DIRECTION('',(0.,1.,0.));
#16047=DIRECTION('center_axis',(-0.342020143325668,0.,0.939692620785909));
#16048=DIRECTION('ref_axis',(0.939692620785909,0.,0.342020143325668));
#16049=DIRECTION('',(-0.939692620785909,0.,-0.342020143325668));
#16050=DIRECTION('',(0.939692620785909,0.,0.342020143325668));
#16051=DIRECTION('',(0.,1.,0.));
#16052=DIRECTION('center_axis',(-1.,0.,0.));
#16053=DIRECTION('ref_axis',(0.,0.,1.));
#16054=DIRECTION('',(0.,0.,-1.));
#16055=DIRECTION('',(0.,0.,1.));
#16056=DIRECTION('',(0.,1.,0.));
#16057=DIRECTION('center_axis',(-0.342020143325668,0.,-0.939692620785909));
#16058=DIRECTION('ref_axis',(-0.939692620785909,0.,0.342020143325668));
#16059=DIRECTION('',(0.939692620785909,0.,-0.342020143325668));
#16060=DIRECTION('',(-0.939692620785909,0.,0.342020143325668));
#16061=DIRECTION('',(0.,1.,0.));
#16062=DIRECTION('center_axis',(-1.,0.,0.));
#16063=DIRECTION('ref_axis',(0.,0.,1.));
#16064=DIRECTION('',(0.,0.,-1.));
#16065=DIRECTION('',(0.,0.,1.));
#16066=DIRECTION('',(0.,1.,0.));
#16067=DIRECTION('center_axis',(-0.342020143325668,0.,0.939692620785909));
#16068=DIRECTION('ref_axis',(0.939692620785909,0.,0.342020143325668));
#16069=DIRECTION('',(-0.939692620785909,0.,-0.342020143325668));
#16070=DIRECTION('',(0.939692620785909,0.,0.342020143325668));
#16071=DIRECTION('',(0.,1.,0.));
#16072=DIRECTION('center_axis',(-1.,0.,0.));
#16073=DIRECTION('ref_axis',(0.,0.,1.));
#16074=DIRECTION('',(0.,0.,-1.));
#16075=DIRECTION('',(0.,0.,1.));
#16076=DIRECTION('',(0.,1.,0.));
#16077=DIRECTION('center_axis',(-0.342020143325668,0.,-0.939692620785909));
#16078=DIRECTION('ref_axis',(-0.939692620785909,0.,0.342020143325668));
#16079=DIRECTION('',(0.939692620785909,0.,-0.342020143325668));
#16080=DIRECTION('',(-0.939692620785909,0.,0.342020143325668));
#16081=DIRECTION('',(0.,1.,0.));
#16082=DIRECTION('center_axis',(-1.,0.,0.));
#16083=DIRECTION('ref_axis',(0.,0.,1.));
#16084=DIRECTION('',(0.,0.,-1.));
#16085=DIRECTION('',(0.,0.,1.));
#16086=DIRECTION('',(0.,1.,0.));
#16087=DIRECTION('center_axis',(-0.342020143325668,0.,0.939692620785909));
#16088=DIRECTION('ref_axis',(0.939692620785909,0.,0.342020143325668));
#16089=DIRECTION('',(-0.939692620785909,0.,-0.342020143325668));
#16090=DIRECTION('',(0.939692620785909,0.,0.342020143325668));
#16091=DIRECTION('',(0.,1.,0.));
#16092=DIRECTION('center_axis',(-1.,0.,0.));
#16093=DIRECTION('ref_axis',(0.,0.,1.));
#16094=DIRECTION('',(0.,0.,-1.));
#16095=DIRECTION('',(0.,0.,1.));
#16096=DIRECTION('',(0.,1.,0.));
#16097=DIRECTION('center_axis',(-0.342020143325668,0.,-0.939692620785909));
#16098=DIRECTION('ref_axis',(-0.939692620785909,0.,0.342020143325668));
#16099=DIRECTION('',(0.939692620785909,0.,-0.342020143325668));
#16100=DIRECTION('',(-0.939692620785909,0.,0.342020143325668));
#16101=DIRECTION('',(0.,1.,0.));
#16102=DIRECTION('center_axis',(-1.,0.,0.));
#16103=DIRECTION('ref_axis',(0.,0.,1.));
#16104=DIRECTION('',(0.,0.,-1.));
#16105=DIRECTION('',(0.,0.,1.));
#16106=DIRECTION('',(0.,1.,0.));
#16107=DIRECTION('center_axis',(-0.342020143325668,0.,0.939692620785909));
#16108=DIRECTION('ref_axis',(0.939692620785909,0.,0.342020143325668));
#16109=DIRECTION('',(-0.939692620785909,0.,-0.342020143325668));
#16110=DIRECTION('',(0.939692620785909,0.,0.342020143325668));
#16111=DIRECTION('',(0.,1.,0.));
#16112=DIRECTION('center_axis',(-1.,0.,0.));
#16113=DIRECTION('ref_axis',(0.,0.,1.));
#16114=DIRECTION('',(0.,0.,-1.));
#16115=DIRECTION('',(0.,0.,1.));
#16116=DIRECTION('',(0.,1.,0.));
#16117=DIRECTION('center_axis',(-0.342020143325668,0.,-0.939692620785909));
#16118=DIRECTION('ref_axis',(-0.939692620785909,0.,0.342020143325668));
#16119=DIRECTION('',(0.939692620785909,0.,-0.342020143325668));
#16120=DIRECTION('',(-0.939692620785909,0.,0.342020143325668));
#16121=DIRECTION('',(0.,1.,0.));
#16122=DIRECTION('center_axis',(-1.,0.,0.));
#16123=DIRECTION('ref_axis',(0.,0.,1.));
#16124=DIRECTION('',(0.,0.,-1.));
#16125=DIRECTION('',(0.,0.,1.));
#16126=DIRECTION('',(0.,1.,0.));
#16127=DIRECTION('center_axis',(-0.342020143325668,0.,0.939692620785909));
#16128=DIRECTION('ref_axis',(0.939692620785909,0.,0.342020143325668));
#16129=DIRECTION('',(-0.939692620785909,0.,-0.342020143325668));
#16130=DIRECTION('',(0.939692620785909,0.,0.342020143325668));
#16131=DIRECTION('',(0.,1.,0.));
#16132=DIRECTION('center_axis',(-1.,0.,0.));
#16133=DIRECTION('ref_axis',(0.,0.,1.));
#16134=DIRECTION('',(0.,0.,-1.));
#16135=DIRECTION('',(0.,0.,1.));
#16136=DIRECTION('',(0.,1.,0.));
#16137=DIRECTION('center_axis',(-0.342020143325668,0.,-0.939692620785909));
#16138=DIRECTION('ref_axis',(-0.939692620785909,0.,0.342020143325668));
#16139=DIRECTION('',(0.939692620785909,0.,-0.342020143325668));
#16140=DIRECTION('',(-0.939692620785909,0.,0.342020143325668));
#16141=DIRECTION('',(0.,1.,0.));
#16142=DIRECTION('center_axis',(-1.,0.,0.));
#16143=DIRECTION('ref_axis',(0.,0.,1.));
#16144=DIRECTION('',(0.,0.,-1.));
#16145=DIRECTION('',(0.,0.,1.));
#16146=DIRECTION('',(0.,1.,0.));
#16147=DIRECTION('center_axis',(-0.342020143325668,0.,0.939692620785909));
#16148=DIRECTION('ref_axis',(0.939692620785909,0.,0.342020143325668));
#16149=DIRECTION('',(-0.939692620785909,0.,-0.342020143325668));
#16150=DIRECTION('',(0.939692620785909,0.,0.342020143325668));
#16151=DIRECTION('',(0.,1.,0.));
#16152=DIRECTION('center_axis',(-1.,0.,0.));
#16153=DIRECTION('ref_axis',(0.,0.,1.));
#16154=DIRECTION('',(0.,0.,-1.));
#16155=DIRECTION('',(0.,0.,1.));
#16156=DIRECTION('',(0.,1.,0.));
#16157=DIRECTION('center_axis',(-0.342020143325668,0.,-0.939692620785909));
#16158=DIRECTION('ref_axis',(-0.939692620785909,0.,0.342020143325668));
#16159=DIRECTION('',(0.939692620785909,0.,-0.342020143325668));
#16160=DIRECTION('',(-0.939692620785909,0.,0.342020143325668));
#16161=DIRECTION('',(0.,1.,0.));
#16162=DIRECTION('center_axis',(-1.,0.,0.));
#16163=DIRECTION('ref_axis',(0.,0.,1.));
#16164=DIRECTION('',(0.,0.,-1.));
#16165=DIRECTION('',(0.,0.,1.));
#16166=DIRECTION('',(0.,1.,0.));
#16167=DIRECTION('center_axis',(-0.342020143325668,0.,0.939692620785909));
#16168=DIRECTION('ref_axis',(0.939692620785909,0.,0.342020143325668));
#16169=DIRECTION('',(-0.939692620785909,0.,-0.342020143325668));
#16170=DIRECTION('',(0.939692620785909,0.,0.342020143325668));
#16171=DIRECTION('',(0.,1.,0.));
#16172=DIRECTION('center_axis',(-1.,0.,0.));
#16173=DIRECTION('ref_axis',(0.,0.,1.));
#16174=DIRECTION('',(0.,0.,-1.));
#16175=DIRECTION('',(0.,0.,1.));
#16176=DIRECTION('',(0.,1.,0.));
#16177=DIRECTION('center_axis',(-0.342020143325668,0.,-0.939692620785909));
#16178=DIRECTION('ref_axis',(-0.939692620785909,0.,0.342020143325668));
#16179=DIRECTION('',(0.939692620785909,0.,-0.342020143325668));
#16180=DIRECTION('',(-0.939692620785909,0.,0.342020143325668));
#16181=DIRECTION('',(0.,1.,0.));
#16182=DIRECTION('center_axis',(-1.,0.,0.));
#16183=DIRECTION('ref_axis',(0.,0.,1.));
#16184=DIRECTION('',(0.,0.,-1.));
#16185=DIRECTION('',(0.,0.,1.));
#16186=DIRECTION('',(0.,1.,0.));
#16187=DIRECTION('center_axis',(-0.342020143325662,0.,0.939692620785911));
#16188=DIRECTION('ref_axis',(0.939692620785911,0.,0.342020143325662));
#16189=DIRECTION('',(-0.939692620785911,0.,-0.342020143325662));
#16190=DIRECTION('',(0.939692620785911,0.,0.342020143325662));
#16191=DIRECTION('',(0.,1.,0.));
#16192=DIRECTION('center_axis',(-1.,0.,0.));
#16193=DIRECTION('ref_axis',(0.,0.,1.));
#16194=DIRECTION('',(0.,0.,-1.));
#16195=DIRECTION('',(0.,0.,1.));
#16196=DIRECTION('',(0.,1.,0.));
#16197=DIRECTION('center_axis',(-0.342020143325662,0.,-0.939692620785911));
#16198=DIRECTION('ref_axis',(-0.939692620785911,0.,0.342020143325662));
#16199=DIRECTION('',(0.939692620785911,0.,-0.342020143325662));
#16200=DIRECTION('',(-0.939692620785911,0.,0.342020143325662));
#16201=DIRECTION('',(0.,1.,0.));
#16202=DIRECTION('center_axis',(-1.,0.,0.));
#16203=DIRECTION('ref_axis',(0.,0.,1.));
#16204=DIRECTION('',(0.,0.,-1.));
#16205=DIRECTION('',(0.,0.,1.));
#16206=DIRECTION('',(0.,1.,0.));
#16207=DIRECTION('center_axis',(-0.342020143325668,0.,0.939692620785909));
#16208=DIRECTION('ref_axis',(0.939692620785909,0.,0.342020143325668));
#16209=DIRECTION('',(-0.939692620785909,0.,-0.342020143325668));
#16210=DIRECTION('',(0.939692620785909,0.,0.342020143325668));
#16211=DIRECTION('',(0.,1.,0.));
#16212=DIRECTION('center_axis',(-1.,0.,0.));
#16213=DIRECTION('ref_axis',(0.,0.,1.));
#16214=DIRECTION('',(0.,0.,-1.));
#16215=DIRECTION('',(0.,0.,1.));
#16216=DIRECTION('',(0.,1.,0.));
#16217=DIRECTION('center_axis',(-0.342020143325668,0.,-0.939692620785909));
#16218=DIRECTION('ref_axis',(-0.939692620785909,0.,0.342020143325668));
#16219=DIRECTION('',(0.939692620785909,0.,-0.342020143325668));
#16220=DIRECTION('',(-0.939692620785909,0.,0.342020143325668));
#16221=DIRECTION('',(0.,1.,0.));
#16222=DIRECTION('center_axis',(-1.,0.,0.));
#16223=DIRECTION('ref_axis',(0.,0.,1.));
#16224=DIRECTION('',(0.,0.,-1.));
#16225=DIRECTION('',(0.,0.,1.));
#16226=DIRECTION('',(0.,1.,0.));
#16227=DIRECTION('center_axis',(-0.342020143325668,0.,0.939692620785909));
#16228=DIRECTION('ref_axis',(0.939692620785909,0.,0.342020143325668));
#16229=DIRECTION('',(-0.939692620785909,0.,-0.342020143325668));
#16230=DIRECTION('',(0.939692620785909,0.,0.342020143325668));
#16231=DIRECTION('',(0.,1.,0.));
#16232=DIRECTION('center_axis',(-1.,0.,0.));
#16233=DIRECTION('ref_axis',(0.,0.,1.));
#16234=DIRECTION('',(0.,0.,-1.));
#16235=DIRECTION('',(0.,0.,1.));
#16236=DIRECTION('',(0.,1.,0.));
#16237=DIRECTION('center_axis',(-0.342020143325668,0.,-0.939692620785909));
#16238=DIRECTION('ref_axis',(-0.939692620785909,0.,0.342020143325668));
#16239=DIRECTION('',(0.939692620785909,0.,-0.342020143325668));
#16240=DIRECTION('',(-0.939692620785909,0.,0.342020143325668));
#16241=DIRECTION('',(0.,1.,0.));
#16242=DIRECTION('center_axis',(-1.,0.,0.));
#16243=DIRECTION('ref_axis',(0.,0.,1.));
#16244=DIRECTION('',(0.,0.,-1.));
#16245=DIRECTION('',(0.,0.,1.));
#16246=DIRECTION('',(0.,1.,0.));
#16247=DIRECTION('center_axis',(-0.342020143325668,0.,0.939692620785909));
#16248=DIRECTION('ref_axis',(0.939692620785909,0.,0.342020143325668));
#16249=DIRECTION('',(-0.939692620785909,0.,-0.342020143325668));
#16250=DIRECTION('',(0.939692620785909,0.,0.342020143325668));
#16251=DIRECTION('',(0.,1.,0.));
#16252=DIRECTION('center_axis',(-1.,0.,0.));
#16253=DIRECTION('ref_axis',(0.,0.,1.));
#16254=DIRECTION('',(0.,0.,-1.));
#16255=DIRECTION('',(0.,0.,1.));
#16256=DIRECTION('',(0.,1.,0.));
#16257=DIRECTION('center_axis',(-0.342020143325662,0.,-0.939692620785911));
#16258=DIRECTION('ref_axis',(-0.939692620785911,0.,0.342020143325662));
#16259=DIRECTION('',(0.939692620785911,0.,-0.342020143325662));
#16260=DIRECTION('',(-0.939692620785911,0.,0.342020143325662));
#16261=DIRECTION('',(0.,1.,0.));
#16262=DIRECTION('center_axis',(-1.,0.,0.));
#16263=DIRECTION('ref_axis',(0.,0.,1.));
#16264=DIRECTION('',(0.,0.,-1.));
#16265=DIRECTION('',(0.,0.,1.));
#16266=DIRECTION('',(0.,1.,0.));
#16267=DIRECTION('center_axis',(-0.342020143325668,0.,0.939692620785909));
#16268=DIRECTION('ref_axis',(0.939692620785909,0.,0.342020143325668));
#16269=DIRECTION('',(-0.939692620785909,0.,-0.342020143325668));
#16270=DIRECTION('',(0.939692620785909,0.,0.342020143325668));
#16271=DIRECTION('',(0.,1.,0.));
#16272=DIRECTION('center_axis',(-1.,0.,0.));
#16273=DIRECTION('ref_axis',(0.,0.,1.));
#16274=DIRECTION('',(0.,0.,-1.));
#16275=DIRECTION('',(0.,0.,1.));
#16276=DIRECTION('',(0.,1.,0.));
#16277=DIRECTION('center_axis',(-0.342020143325668,0.,-0.939692620785909));
#16278=DIRECTION('ref_axis',(-0.939692620785909,0.,0.342020143325668));
#16279=DIRECTION('',(0.939692620785909,0.,-0.342020143325668));
#16280=DIRECTION('',(-0.939692620785909,0.,0.342020143325668));
#16281=DIRECTION('',(0.,1.,0.));
#16282=DIRECTION('center_axis',(-1.,0.,0.));
#16283=DIRECTION('ref_axis',(0.,0.,1.));
#16284=DIRECTION('',(0.,0.,-1.));
#16285=DIRECTION('',(0.,0.,1.));
#16286=DIRECTION('',(0.,1.,0.));
#16287=DIRECTION('center_axis',(-0.342020143325662,0.,0.939692620785911));
#16288=DIRECTION('ref_axis',(0.939692620785911,0.,0.342020143325662));
#16289=DIRECTION('',(-0.939692620785911,0.,-0.342020143325662));
#16290=DIRECTION('',(0.939692620785911,0.,0.342020143325662));
#16291=DIRECTION('',(0.,1.,0.));
#16292=DIRECTION('center_axis',(-1.,0.,0.));
#16293=DIRECTION('ref_axis',(0.,0.,1.));
#16294=DIRECTION('',(0.,0.,-1.));
#16295=DIRECTION('',(0.,0.,1.));
#16296=DIRECTION('',(0.,1.,0.));
#16297=DIRECTION('center_axis',(-0.342020143325668,0.,-0.939692620785909));
#16298=DIRECTION('ref_axis',(-0.939692620785909,0.,0.342020143325668));
#16299=DIRECTION('',(0.939692620785909,0.,-0.342020143325668));
#16300=DIRECTION('',(-0.939692620785909,0.,0.342020143325668));
#16301=DIRECTION('',(0.,1.,0.));
#16302=DIRECTION('center_axis',(-1.,0.,0.));
#16303=DIRECTION('ref_axis',(0.,0.,1.));
#16304=DIRECTION('',(0.,0.,-1.));
#16305=DIRECTION('',(0.,0.,1.));
#16306=DIRECTION('',(0.,1.,0.));
#16307=DIRECTION('center_axis',(-0.342020143325668,0.,0.939692620785909));
#16308=DIRECTION('ref_axis',(0.939692620785909,0.,0.342020143325668));
#16309=DIRECTION('',(-0.939692620785909,0.,-0.342020143325668));
#16310=DIRECTION('',(0.939692620785909,0.,0.342020143325668));
#16311=DIRECTION('',(0.,1.,0.));
#16312=DIRECTION('center_axis',(-1.,0.,0.));
#16313=DIRECTION('ref_axis',(0.,0.,1.));
#16314=DIRECTION('',(0.,0.,-1.));
#16315=DIRECTION('',(0.,0.,1.));
#16316=DIRECTION('',(0.,1.,0.));
#16317=DIRECTION('center_axis',(-0.342020143325668,0.,-0.939692620785909));
#16318=DIRECTION('ref_axis',(-0.939692620785909,0.,0.342020143325668));
#16319=DIRECTION('',(0.939692620785909,0.,-0.342020143325668));
#16320=DIRECTION('',(-0.939692620785909,0.,0.342020143325668));
#16321=DIRECTION('',(0.,1.,0.));
#16322=DIRECTION('center_axis',(-1.,0.,0.));
#16323=DIRECTION('ref_axis',(0.,0.,1.));
#16324=DIRECTION('',(0.,0.,-1.));
#16325=DIRECTION('',(0.,0.,1.));
#16326=DIRECTION('',(0.,1.,0.));
#16327=DIRECTION('center_axis',(-0.342020143325668,0.,0.939692620785909));
#16328=DIRECTION('ref_axis',(0.939692620785909,0.,0.342020143325668));
#16329=DIRECTION('',(-0.939692620785909,0.,-0.342020143325668));
#16330=DIRECTION('',(0.939692620785909,0.,0.342020143325668));
#16331=DIRECTION('',(0.,1.,0.));
#16332=DIRECTION('center_axis',(-1.,0.,0.));
#16333=DIRECTION('ref_axis',(0.,0.,1.));
#16334=DIRECTION('',(0.,0.,-1.));
#16335=DIRECTION('',(0.,0.,1.));
#16336=DIRECTION('',(0.,1.,0.));
#16337=DIRECTION('center_axis',(-0.342020143325662,0.,-0.939692620785911));
#16338=DIRECTION('ref_axis',(-0.939692620785911,0.,0.342020143325662));
#16339=DIRECTION('',(0.939692620785911,0.,-0.342020143325662));
#16340=DIRECTION('',(-0.939692620785911,0.,0.342020143325662));
#16341=DIRECTION('',(0.,1.,0.));
#16342=DIRECTION('center_axis',(-1.,0.,0.));
#16343=DIRECTION('ref_axis',(0.,0.,1.));
#16344=DIRECTION('',(0.,0.,-1.));
#16345=DIRECTION('',(0.,0.,1.));
#16346=DIRECTION('',(0.,1.,0.));
#16347=DIRECTION('center_axis',(-0.342020143325668,0.,0.939692620785909));
#16348=DIRECTION('ref_axis',(0.939692620785909,0.,0.342020143325668));
#16349=DIRECTION('',(-0.939692620785909,0.,-0.342020143325668));
#16350=DIRECTION('',(0.939692620785909,0.,0.342020143325668));
#16351=DIRECTION('',(0.,1.,0.));
#16352=DIRECTION('center_axis',(-1.,0.,0.));
#16353=DIRECTION('ref_axis',(0.,0.,1.));
#16354=DIRECTION('',(0.,0.,-1.));
#16355=DIRECTION('',(0.,0.,1.));
#16356=DIRECTION('',(0.,1.,0.));
#16357=DIRECTION('center_axis',(-0.342020143325668,0.,-0.939692620785909));
#16358=DIRECTION('ref_axis',(-0.939692620785909,0.,0.342020143325668));
#16359=DIRECTION('',(0.939692620785909,0.,-0.342020143325668));
#16360=DIRECTION('',(-0.939692620785909,0.,0.342020143325668));
#16361=DIRECTION('',(0.,1.,0.));
#16362=DIRECTION('center_axis',(-1.,0.,0.));
#16363=DIRECTION('ref_axis',(0.,0.,1.));
#16364=DIRECTION('',(0.,0.,-1.));
#16365=DIRECTION('',(0.,0.,1.));
#16366=DIRECTION('',(0.,1.,0.));
#16367=DIRECTION('center_axis',(-0.342020143325668,0.,0.939692620785909));
#16368=DIRECTION('ref_axis',(0.939692620785909,0.,0.342020143325668));
#16369=DIRECTION('',(-0.939692620785909,0.,-0.342020143325668));
#16370=DIRECTION('',(0.939692620785909,0.,0.342020143325668));
#16371=DIRECTION('',(0.,1.,0.));
#16372=DIRECTION('center_axis',(-1.,0.,0.));
#16373=DIRECTION('ref_axis',(0.,0.,1.));
#16374=DIRECTION('',(0.,0.,-1.));
#16375=DIRECTION('',(0.,0.,1.));
#16376=DIRECTION('',(0.,1.,0.));
#16377=DIRECTION('center_axis',(-0.342020143325668,0.,-0.939692620785909));
#16378=DIRECTION('ref_axis',(-0.939692620785909,0.,0.342020143325668));
#16379=DIRECTION('',(0.939692620785909,0.,-0.342020143325668));
#16380=DIRECTION('',(-0.939692620785909,0.,0.342020143325668));
#16381=DIRECTION('',(0.,1.,0.));
#16382=DIRECTION('center_axis',(-1.,0.,0.));
#16383=DIRECTION('ref_axis',(0.,0.,1.));
#16384=DIRECTION('',(0.,0.,-1.));
#16385=DIRECTION('',(0.,0.,1.));
#16386=DIRECTION('',(0.,1.,0.));
#16387=DIRECTION('center_axis',(-0.342020143325668,0.,0.939692620785909));
#16388=DIRECTION('ref_axis',(0.939692620785909,0.,0.342020143325668));
#16389=DIRECTION('',(-0.939692620785909,0.,-0.342020143325668));
#16390=DIRECTION('',(0.939692620785909,0.,0.342020143325668));
#16391=DIRECTION('',(0.,1.,0.));
#16392=DIRECTION('center_axis',(-1.,0.,0.));
#16393=DIRECTION('ref_axis',(0.,0.,1.));
#16394=DIRECTION('',(0.,0.,-1.));
#16395=DIRECTION('',(0.,0.,1.));
#16396=DIRECTION('',(0.,1.,0.));
#16397=DIRECTION('center_axis',(-0.342020143325668,0.,-0.939692620785909));
#16398=DIRECTION('ref_axis',(-0.939692620785909,0.,0.342020143325668));
#16399=DIRECTION('',(0.939692620785909,0.,-0.342020143325668));
#16400=DIRECTION('',(-0.939692620785909,0.,0.342020143325668));
#16401=DIRECTION('',(0.,1.,0.));
#16402=DIRECTION('center_axis',(-1.,0.,0.));
#16403=DIRECTION('ref_axis',(0.,0.,1.));
#16404=DIRECTION('',(0.,0.,-1.));
#16405=DIRECTION('',(0.,0.,1.));
#16406=DIRECTION('',(0.,1.,0.));
#16407=DIRECTION('center_axis',(-0.342020143325668,0.,0.939692620785909));
#16408=DIRECTION('ref_axis',(0.939692620785909,0.,0.342020143325668));
#16409=DIRECTION('',(-0.939692620785909,0.,-0.342020143325668));
#16410=DIRECTION('',(0.939692620785909,0.,0.342020143325668));
#16411=DIRECTION('',(0.,1.,0.));
#16412=DIRECTION('center_axis',(-1.,0.,0.));
#16413=DIRECTION('ref_axis',(0.,0.,1.));
#16414=DIRECTION('',(0.,0.,-1.));
#16415=DIRECTION('',(0.,0.,1.));
#16416=DIRECTION('',(0.,1.,0.));
#16417=DIRECTION('center_axis',(-0.342020143325662,0.,-0.939692620785911));
#16418=DIRECTION('ref_axis',(-0.939692620785911,0.,0.342020143325662));
#16419=DIRECTION('',(0.939692620785911,0.,-0.342020143325662));
#16420=DIRECTION('',(-0.939692620785911,0.,0.342020143325662));
#16421=DIRECTION('',(0.,1.,0.));
#16422=DIRECTION('center_axis',(-1.,0.,0.));
#16423=DIRECTION('ref_axis',(0.,0.,1.));
#16424=DIRECTION('',(0.,0.,-1.));
#16425=DIRECTION('',(0.,0.,1.));
#16426=DIRECTION('',(0.,1.,0.));
#16427=DIRECTION('center_axis',(-0.342020143325668,0.,0.939692620785909));
#16428=DIRECTION('ref_axis',(0.939692620785909,0.,0.342020143325668));
#16429=DIRECTION('',(-0.939692620785909,0.,-0.342020143325668));
#16430=DIRECTION('',(0.939692620785909,0.,0.342020143325668));
#16431=DIRECTION('',(0.,1.,0.));
#16432=DIRECTION('center_axis',(-1.,0.,0.));
#16433=DIRECTION('ref_axis',(0.,0.,1.));
#16434=DIRECTION('',(0.,0.,-1.));
#16435=DIRECTION('',(0.,0.,1.));
#16436=DIRECTION('',(0.,1.,0.));
#16437=DIRECTION('center_axis',(-0.342020143325668,0.,-0.939692620785909));
#16438=DIRECTION('ref_axis',(-0.939692620785909,0.,0.342020143325668));
#16439=DIRECTION('',(0.939692620785909,0.,-0.342020143325668));
#16440=DIRECTION('',(-0.939692620785909,0.,0.342020143325668));
#16441=DIRECTION('',(0.,1.,0.));
#16442=DIRECTION('center_axis',(-1.,0.,0.));
#16443=DIRECTION('ref_axis',(0.,0.,1.));
#16444=DIRECTION('',(0.,0.,-1.));
#16445=DIRECTION('',(0.,0.,1.));
#16446=DIRECTION('',(0.,1.,0.));
#16447=DIRECTION('center_axis',(-0.342020143325662,0.,0.939692620785911));
#16448=DIRECTION('ref_axis',(0.939692620785911,0.,0.342020143325662));
#16449=DIRECTION('',(-0.939692620785911,0.,-0.342020143325662));
#16450=DIRECTION('',(0.939692620785911,0.,0.342020143325662));
#16451=DIRECTION('',(0.,1.,0.));
#16452=DIRECTION('center_axis',(-1.,0.,0.));
#16453=DIRECTION('ref_axis',(0.,0.,1.));
#16454=DIRECTION('',(0.,0.,-1.));
#16455=DIRECTION('',(0.,0.,1.));
#16456=DIRECTION('',(0.,1.,0.));
#16457=DIRECTION('center_axis',(-0.342020143325668,0.,-0.939692620785909));
#16458=DIRECTION('ref_axis',(-0.939692620785909,0.,0.342020143325668));
#16459=DIRECTION('',(0.939692620785909,0.,-0.342020143325668));
#16460=DIRECTION('',(-0.939692620785909,0.,0.342020143325668));
#16461=DIRECTION('',(0.,1.,0.));
#16462=DIRECTION('center_axis',(-1.,0.,0.));
#16463=DIRECTION('ref_axis',(0.,0.,1.));
#16464=DIRECTION('',(0.,0.,-1.));
#16465=DIRECTION('',(0.,0.,1.));
#16466=DIRECTION('',(0.,1.,0.));
#16467=DIRECTION('center_axis',(-0.342020143325668,0.,0.939692620785909));
#16468=DIRECTION('ref_axis',(0.939692620785909,0.,0.342020143325668));
#16469=DIRECTION('',(-0.939692620785909,0.,-0.342020143325668));
#16470=DIRECTION('',(0.939692620785909,0.,0.342020143325668));
#16471=DIRECTION('',(0.,1.,0.));
#16472=DIRECTION('center_axis',(-1.,0.,0.));
#16473=DIRECTION('ref_axis',(0.,0.,1.));
#16474=DIRECTION('',(0.,0.,-1.));
#16475=DIRECTION('',(0.,0.,1.));
#16476=DIRECTION('',(0.,1.,0.));
#16477=DIRECTION('center_axis',(-0.342020143325668,0.,-0.939692620785909));
#16478=DIRECTION('ref_axis',(-0.939692620785909,0.,0.342020143325668));
#16479=DIRECTION('',(0.939692620785909,0.,-0.342020143325668));
#16480=DIRECTION('',(-0.939692620785909,0.,0.342020143325668));
#16481=DIRECTION('',(0.,1.,0.));
#16482=DIRECTION('center_axis',(-1.,0.,0.));
#16483=DIRECTION('ref_axis',(0.,0.,1.));
#16484=DIRECTION('',(0.,0.,-1.));
#16485=DIRECTION('',(0.,0.,1.));
#16486=DIRECTION('',(0.,1.,0.));
#16487=DIRECTION('center_axis',(-0.342020143325668,0.,0.939692620785909));
#16488=DIRECTION('ref_axis',(0.939692620785909,0.,0.342020143325668));
#16489=DIRECTION('',(-0.939692620785909,0.,-0.342020143325668));
#16490=DIRECTION('',(0.939692620785909,0.,0.342020143325668));
#16491=DIRECTION('',(0.,1.,0.));
#16492=DIRECTION('center_axis',(-1.,0.,0.));
#16493=DIRECTION('ref_axis',(0.,0.,1.));
#16494=DIRECTION('',(0.,0.,-1.));
#16495=DIRECTION('',(0.,0.,1.));
#16496=DIRECTION('',(0.,1.,0.));
#16497=DIRECTION('center_axis',(-0.342020143325662,0.,-0.939692620785911));
#16498=DIRECTION('ref_axis',(-0.939692620785911,0.,0.342020143325662));
#16499=DIRECTION('',(0.939692620785911,0.,-0.342020143325662));
#16500=DIRECTION('',(-0.939692620785911,0.,0.342020143325662));
#16501=DIRECTION('',(0.,1.,0.));
#16502=DIRECTION('center_axis',(-1.,0.,0.));
#16503=DIRECTION('ref_axis',(0.,0.,1.));
#16504=DIRECTION('',(0.,0.,-1.));
#16505=DIRECTION('',(0.,0.,1.));
#16506=DIRECTION('',(0.,1.,0.));
#16507=DIRECTION('center_axis',(-0.342020143325668,0.,0.939692620785909));
#16508=DIRECTION('ref_axis',(0.939692620785909,0.,0.342020143325668));
#16509=DIRECTION('',(-0.939692620785909,0.,-0.342020143325668));
#16510=DIRECTION('',(0.939692620785909,0.,0.342020143325668));
#16511=DIRECTION('',(0.,1.,0.));
#16512=DIRECTION('center_axis',(-1.,0.,0.));
#16513=DIRECTION('ref_axis',(0.,0.,1.));
#16514=DIRECTION('',(0.,0.,-1.));
#16515=DIRECTION('',(0.,0.,1.));
#16516=DIRECTION('',(0.,1.,0.));
#16517=DIRECTION('center_axis',(-0.342020143325668,0.,-0.939692620785909));
#16518=DIRECTION('ref_axis',(-0.939692620785909,0.,0.342020143325668));
#16519=DIRECTION('',(0.939692620785909,0.,-0.342020143325668));
#16520=DIRECTION('',(-0.939692620785909,0.,0.342020143325668));
#16521=DIRECTION('',(0.,1.,0.));
#16522=DIRECTION('center_axis',(-1.,0.,0.));
#16523=DIRECTION('ref_axis',(0.,0.,1.));
#16524=DIRECTION('',(0.,0.,-1.));
#16525=DIRECTION('',(0.,0.,1.));
#16526=DIRECTION('',(0.,1.,0.));
#16527=DIRECTION('center_axis',(-0.342020143325668,0.,0.939692620785909));
#16528=DIRECTION('ref_axis',(0.939692620785909,0.,0.342020143325668));
#16529=DIRECTION('',(-0.939692620785909,0.,-0.342020143325668));
#16530=DIRECTION('',(0.939692620785909,0.,0.342020143325668));
#16531=DIRECTION('',(0.,1.,0.));
#16532=DIRECTION('center_axis',(-1.,0.,0.));
#16533=DIRECTION('ref_axis',(0.,0.,1.));
#16534=DIRECTION('',(0.,0.,-1.));
#16535=DIRECTION('',(0.,0.,1.));
#16536=DIRECTION('',(0.,1.,0.));
#16537=DIRECTION('center_axis',(-0.342020143325668,0.,-0.939692620785909));
#16538=DIRECTION('ref_axis',(-0.939692620785909,0.,0.342020143325668));
#16539=DIRECTION('',(0.939692620785909,0.,-0.342020143325668));
#16540=DIRECTION('',(-0.939692620785909,0.,0.342020143325668));
#16541=DIRECTION('',(0.,1.,0.));
#16542=DIRECTION('center_axis',(-1.,0.,0.));
#16543=DIRECTION('ref_axis',(0.,0.,1.));
#16544=DIRECTION('',(0.,0.,-1.));
#16545=DIRECTION('',(0.,0.,1.));
#16546=DIRECTION('',(0.,1.,0.));
#16547=DIRECTION('center_axis',(-0.342020143325668,0.,0.939692620785909));
#16548=DIRECTION('ref_axis',(0.939692620785909,0.,0.342020143325668));
#16549=DIRECTION('',(-0.939692620785909,0.,-0.342020143325668));
#16550=DIRECTION('',(0.939692620785909,0.,0.342020143325668));
#16551=DIRECTION('',(0.,1.,0.));
#16552=DIRECTION('center_axis',(-1.,0.,0.));
#16553=DIRECTION('ref_axis',(0.,0.,1.));
#16554=DIRECTION('',(0.,0.,-1.));
#16555=DIRECTION('',(0.,0.,1.));
#16556=DIRECTION('',(0.,1.,0.));
#16557=DIRECTION('center_axis',(-0.342020143325665,0.,-0.93969262078591));
#16558=DIRECTION('ref_axis',(-0.93969262078591,0.,0.342020143325665));
#16559=DIRECTION('',(0.93969262078591,0.,-0.342020143325665));
#16560=DIRECTION('',(-0.93969262078591,0.,0.342020143325665));
#16561=DIRECTION('',(0.,1.,0.));
#16562=DIRECTION('center_axis',(-1.,0.,0.));
#16563=DIRECTION('ref_axis',(0.,0.,1.));
#16564=DIRECTION('',(0.,0.,-1.));
#16565=DIRECTION('',(0.,0.,1.));
#16566=DIRECTION('',(0.,1.,0.));
#16567=DIRECTION('center_axis',(-0.342020143325668,0.,0.939692620785909));
#16568=DIRECTION('ref_axis',(0.939692620785909,0.,0.342020143325668));
#16569=DIRECTION('',(-0.939692620785909,0.,-0.342020143325668));
#16570=DIRECTION('',(0.939692620785909,0.,0.342020143325668));
#16571=DIRECTION('',(0.,1.,0.));
#16572=DIRECTION('center_axis',(-1.,0.,0.));
#16573=DIRECTION('ref_axis',(0.,0.,1.));
#16574=DIRECTION('',(0.,0.,-1.));
#16575=DIRECTION('',(0.,0.,1.));
#16576=DIRECTION('',(0.,1.,0.));
#16577=DIRECTION('center_axis',(-0.342020143325668,0.,-0.939692620785909));
#16578=DIRECTION('ref_axis',(-0.939692620785909,0.,0.342020143325668));
#16579=DIRECTION('',(0.939692620785909,0.,-0.342020143325668));
#16580=DIRECTION('',(-0.939692620785909,0.,0.342020143325668));
#16581=DIRECTION('',(0.,1.,0.));
#16582=DIRECTION('center_axis',(-1.,0.,0.));
#16583=DIRECTION('ref_axis',(0.,0.,1.));
#16584=DIRECTION('',(0.,0.,-1.));
#16585=DIRECTION('',(0.,0.,1.));
#16586=DIRECTION('',(0.,1.,0.));
#16587=DIRECTION('center_axis',(-0.342020143325665,0.,0.93969262078591));
#16588=DIRECTION('ref_axis',(0.93969262078591,0.,0.342020143325665));
#16589=DIRECTION('',(-0.93969262078591,0.,-0.342020143325665));
#16590=DIRECTION('',(0.93969262078591,0.,0.342020143325665));
#16591=DIRECTION('',(0.,1.,0.));
#16592=DIRECTION('center_axis',(-1.,0.,0.));
#16593=DIRECTION('ref_axis',(0.,0.,1.));
#16594=DIRECTION('',(0.,0.,-1.));
#16595=DIRECTION('',(0.,0.,1.));
#16596=DIRECTION('',(0.,1.,0.));
#16597=DIRECTION('center_axis',(-0.342020143325665,0.,-0.93969262078591));
#16598=DIRECTION('ref_axis',(-0.93969262078591,0.,0.342020143325665));
#16599=DIRECTION('',(0.93969262078591,0.,-0.342020143325665));
#16600=DIRECTION('',(-0.93969262078591,0.,0.342020143325665));
#16601=DIRECTION('',(0.,1.,0.));
#16602=DIRECTION('center_axis',(-1.,0.,0.));
#16603=DIRECTION('ref_axis',(0.,0.,1.));
#16604=DIRECTION('',(0.,0.,-1.));
#16605=DIRECTION('',(0.,0.,1.));
#16606=DIRECTION('',(0.,1.,0.));
#16607=DIRECTION('center_axis',(-0.342020143325668,0.,0.939692620785909));
#16608=DIRECTION('ref_axis',(0.939692620785909,0.,0.342020143325668));
#16609=DIRECTION('',(-0.939692620785909,0.,-0.342020143325668));
#16610=DIRECTION('',(0.939692620785909,0.,0.342020143325668));
#16611=DIRECTION('',(0.,1.,0.));
#16612=DIRECTION('center_axis',(-1.,0.,0.));
#16613=DIRECTION('ref_axis',(0.,0.,1.));
#16614=DIRECTION('',(0.,0.,-1.));
#16615=DIRECTION('',(0.,0.,1.));
#16616=DIRECTION('',(0.,1.,0.));
#16617=DIRECTION('center_axis',(-0.342020143325668,0.,-0.939692620785909));
#16618=DIRECTION('ref_axis',(-0.939692620785909,0.,0.342020143325668));
#16619=DIRECTION('',(0.939692620785909,0.,-0.342020143325668));
#16620=DIRECTION('',(-0.939692620785909,0.,0.342020143325668));
#16621=DIRECTION('',(0.,1.,0.));
#16622=DIRECTION('center_axis',(-1.,0.,0.));
#16623=DIRECTION('ref_axis',(0.,0.,1.));
#16624=DIRECTION('',(0.,0.,-1.));
#16625=DIRECTION('',(0.,0.,1.));
#16626=DIRECTION('',(0.,1.,0.));
#16627=DIRECTION('center_axis',(-0.342020143325668,0.,0.939692620785909));
#16628=DIRECTION('ref_axis',(0.939692620785909,0.,0.342020143325668));
#16629=DIRECTION('',(-0.939692620785909,0.,-0.342020143325668));
#16630=DIRECTION('',(0.939692620785909,0.,0.342020143325668));
#16631=DIRECTION('',(0.,1.,0.));
#16632=DIRECTION('center_axis',(-1.,0.,0.));
#16633=DIRECTION('ref_axis',(0.,0.,1.));
#16634=DIRECTION('',(0.,0.,-1.));
#16635=DIRECTION('',(0.,0.,1.));
#16636=DIRECTION('',(0.,1.,0.));
#16637=DIRECTION('center_axis',(-0.342020143325665,0.,-0.93969262078591));
#16638=DIRECTION('ref_axis',(-0.93969262078591,0.,0.342020143325665));
#16639=DIRECTION('',(0.93969262078591,0.,-0.342020143325665));
#16640=DIRECTION('',(-0.93969262078591,0.,0.342020143325665));
#16641=DIRECTION('',(0.,1.,0.));
#16642=DIRECTION('center_axis',(-1.,0.,0.));
#16643=DIRECTION('ref_axis',(0.,0.,1.));
#16644=DIRECTION('',(0.,0.,-1.));
#16645=DIRECTION('',(0.,0.,1.));
#16646=DIRECTION('',(0.,1.,0.));
#16647=DIRECTION('center_axis',(-0.342020143325668,0.,0.939692620785909));
#16648=DIRECTION('ref_axis',(0.939692620785909,0.,0.342020143325668));
#16649=DIRECTION('',(-0.939692620785909,0.,-0.342020143325668));
#16650=DIRECTION('',(0.939692620785909,0.,0.342020143325668));
#16651=DIRECTION('',(0.,1.,0.));
#16652=DIRECTION('center_axis',(-1.,0.,0.));
#16653=DIRECTION('ref_axis',(0.,0.,1.));
#16654=DIRECTION('',(0.,0.,-1.));
#16655=DIRECTION('',(0.,0.,1.));
#16656=DIRECTION('',(0.,1.,0.));
#16657=DIRECTION('center_axis',(-0.342020143325671,0.,-0.939692620785907));
#16658=DIRECTION('ref_axis',(-0.939692620785907,0.,0.342020143325671));
#16659=DIRECTION('',(0.939692620785907,0.,-0.342020143325671));
#16660=DIRECTION('',(-0.939692620785907,0.,0.342020143325671));
#16661=DIRECTION('',(0.,1.,0.));
#16662=DIRECTION('center_axis',(-1.,0.,0.));
#16663=DIRECTION('ref_axis',(0.,0.,1.));
#16664=DIRECTION('',(0.,0.,-1.));
#16665=DIRECTION('',(0.,0.,1.));
#16666=DIRECTION('',(0.,1.,0.));
#16667=DIRECTION('center_axis',(-0.342020143325668,0.,0.939692620785909));
#16668=DIRECTION('ref_axis',(0.939692620785909,0.,0.342020143325668));
#16669=DIRECTION('',(-0.939692620785909,0.,-0.342020143325668));
#16670=DIRECTION('',(0.939692620785909,0.,0.342020143325668));
#16671=DIRECTION('',(0.,1.,0.));
#16672=DIRECTION('center_axis',(-1.,0.,0.));
#16673=DIRECTION('ref_axis',(0.,0.,1.));
#16674=DIRECTION('',(0.,0.,-1.));
#16675=DIRECTION('',(0.,0.,1.));
#16676=DIRECTION('',(0.,1.,0.));
#16677=DIRECTION('center_axis',(-0.342020143325668,0.,-0.939692620785909));
#16678=DIRECTION('ref_axis',(-0.939692620785909,0.,0.342020143325668));
#16679=DIRECTION('',(0.939692620785909,0.,-0.342020143325668));
#16680=DIRECTION('',(-0.939692620785909,0.,0.342020143325668));
#16681=DIRECTION('',(0.,1.,0.));
#16682=DIRECTION('center_axis',(-1.,0.,0.));
#16683=DIRECTION('ref_axis',(0.,0.,1.));
#16684=DIRECTION('',(0.,0.,-1.));
#16685=DIRECTION('',(0.,0.,1.));
#16686=DIRECTION('',(0.,1.,0.));
#16687=DIRECTION('center_axis',(-0.342020143325668,0.,0.939692620785909));
#16688=DIRECTION('ref_axis',(0.939692620785909,0.,0.342020143325668));
#16689=DIRECTION('',(-0.939692620785909,0.,-0.342020143325668));
#16690=DIRECTION('',(0.939692620785909,0.,0.342020143325668));
#16691=DIRECTION('',(0.,1.,0.));
#16692=DIRECTION('center_axis',(-1.,0.,0.));
#16693=DIRECTION('ref_axis',(0.,0.,1.));
#16694=DIRECTION('',(0.,0.,-1.));
#16695=DIRECTION('',(0.,0.,1.));
#16696=DIRECTION('',(0.,1.,0.));
#16697=DIRECTION('center_axis',(-0.342020143325671,0.,-0.939692620785907));
#16698=DIRECTION('ref_axis',(-0.939692620785907,0.,0.342020143325671));
#16699=DIRECTION('',(0.939692620785907,0.,-0.342020143325671));
#16700=DIRECTION('',(-0.939692620785907,0.,0.342020143325671));
#16701=DIRECTION('',(0.,1.,0.));
#16702=DIRECTION('center_axis',(-1.,0.,0.));
#16703=DIRECTION('ref_axis',(0.,0.,1.));
#16704=DIRECTION('',(0.,0.,-1.));
#16705=DIRECTION('',(0.,0.,1.));
#16706=DIRECTION('center_axis',(0.,1.,0.));
#16707=DIRECTION('ref_axis',(0.,0.,1.));
#16708=DIRECTION('center_axis',(0.,1.,0.));
#16709=DIRECTION('ref_axis',(1.,0.,0.));
#16710=DIRECTION('center_axis',(0.,0.,1.));
#16711=DIRECTION('ref_axis',(1.,0.,0.));
#16712=DIRECTION('center_axis',(0.,0.,1.));
#16713=DIRECTION('ref_axis',(1.,0.,0.));
#16714=DIRECTION('',(0.,0.,-1.));
#16715=DIRECTION('',(0.,0.,-1.));
#16716=DIRECTION('center_axis',(0.,0.,1.));
#16717=DIRECTION('ref_axis',(1.,0.,0.));
#16718=DIRECTION('center_axis',(0.,0.,1.));
#16719=DIRECTION('ref_axis',(1.,0.,0.));
#16720=DIRECTION('center_axis',(0.,0.,1.));
#16721=DIRECTION('ref_axis',(1.,0.,0.));
#19757=CARTESIAN_POINT('',(0.,0.,0.));
#19758=CARTESIAN_POINT('Origin',(1.,0.,10.7));
#19759=CARTESIAN_POINT('',(0.575,-5.20474889637625E-17,10.8));
#19760=CARTESIAN_POINT('Origin',(1.,0.,10.8));
#19761=CARTESIAN_POINT('',(0.575,-5.20474889637625E-17,12.));
#19762=CARTESIAN_POINT('',(0.575,-5.20474889637625E-17,10.7));
#19763=CARTESIAN_POINT('Origin',(1.,0.,12.));
#19764=CARTESIAN_POINT('Origin',(1.,0.,12.));
#19765=CARTESIAN_POINT('Origin',(0.2,-1.,37.));
#19766=CARTESIAN_POINT('',(0.2,-0.6,37.));
#19767=CARTESIAN_POINT('',(0.2,-0.6,11.));
#19768=CARTESIAN_POINT('',(0.2,-0.6,10.8));
#19769=CARTESIAN_POINT('',(0.2,-1.,37.));
#19770=CARTESIAN_POINT('',(0.2,-1.,37.));
#19771=CARTESIAN_POINT('',(0.2,-1.,11.));
#19772=CARTESIAN_POINT('',(0.2,-1.,11.));
#19773=CARTESIAN_POINT('',(0.2,-1.,11.));
#19774=CARTESIAN_POINT('Origin',(0.2,-1.,37.));
#19775=CARTESIAN_POINT('',(0.2,0.6,11.));
#19776=CARTESIAN_POINT('',(0.2,0.6,37.));
#19777=CARTESIAN_POINT('',(0.2,0.6,10.8));
#19778=CARTESIAN_POINT('',(0.2,1.,11.));
#19779=CARTESIAN_POINT('',(0.2,-1.,11.));
#19780=CARTESIAN_POINT('',(0.2,1.,37.));
#19781=CARTESIAN_POINT('',(0.2,1.,11.));
#19782=CARTESIAN_POINT('',(0.2,-1.,37.));
#19783=CARTESIAN_POINT('Origin',(0.2,-1.,11.));
#19784=CARTESIAN_POINT('',(0.,-1.22464679914735E-16,11.));
#19785=CARTESIAN_POINT('Origin',(1.,0.,11.));
#19786=CARTESIAN_POINT('',(-1.,-1.,11.));
#19787=CARTESIAN_POINT('',(-1.,-1.,11.));
#19788=CARTESIAN_POINT('',(-1.,1.,11.));
#19789=CARTESIAN_POINT('',(-1.,-1.,11.));
#19790=CARTESIAN_POINT('',(-1.,1.,11.));
#19791=CARTESIAN_POINT('Origin',(1.,0.,11.));
#19792=CARTESIAN_POINT('Origin',(-1.,-1.,37.));
#19793=CARTESIAN_POINT('',(0.,-1.22464679914735E-16,37.));
#19794=CARTESIAN_POINT('Origin',(1.,0.,37.));
#19795=CARTESIAN_POINT('',(-1.,1.,37.));
#19796=CARTESIAN_POINT('',(0.2,1.,37.));
#19797=CARTESIAN_POINT('',(-1.,-1.,37.));
#19798=CARTESIAN_POINT('',(-1.,-1.,37.));
#19799=CARTESIAN_POINT('',(0.2,-1.,37.));
#19800=CARTESIAN_POINT('Origin',(1.,0.,37.));
#19801=CARTESIAN_POINT('Origin',(-1.,-1.,36.269194724554));
#19802=CARTESIAN_POINT('',(-1.,-1.,36.269194724554));
#19803=CARTESIAN_POINT('',(-1.,-1.,37.));
#19804=CARTESIAN_POINT('',(-1.,1.,36.269194724554));
#19805=CARTESIAN_POINT('',(-1.,1.,37.));
#19806=CARTESIAN_POINT('',(-1.,-1.,36.269194724554));
#19807=CARTESIAN_POINT('Origin',(-1.45,-1.,36.1054081191342));
#19808=CARTESIAN_POINT('',(-1.45,-1.,36.1054081191342));
#19809=CARTESIAN_POINT('',(-1.,-1.,36.269194724554));
#19810=CARTESIAN_POINT('',(-1.45,1.,36.1054081191342));
#19811=CARTESIAN_POINT('',(-1.,1.,36.269194724554));
#19812=CARTESIAN_POINT('',(-1.45,-1.,36.1054081191342));
#19813=CARTESIAN_POINT('Origin',(-1.45,-1.,35.9388369474817));
#19814=CARTESIAN_POINT('',(-1.45,-1.,35.9388369474817));
#19815=CARTESIAN_POINT('',(-1.45,-1.,36.1054081191342));
#19816=CARTESIAN_POINT('',(-1.45,1.,35.9388369474817));
#19817=CARTESIAN_POINT('',(-1.45,1.,36.1054081191342));
#19818=CARTESIAN_POINT('',(-1.45,-1.,35.9388369474817));
#19819=CARTESIAN_POINT('Origin',(-1.,-1.,35.7750503420619));
#19820=CARTESIAN_POINT('',(-1.,-1.,35.7750503420619));
#19821=CARTESIAN_POINT('',(-1.45,-1.,35.9388369474817));
#19822=CARTESIAN_POINT('',(-1.,1.,35.7750503420619));
#19823=CARTESIAN_POINT('',(-1.45,1.,35.9388369474817));
#19824=CARTESIAN_POINT('',(-1.,-1.,35.7750503420619));
#19825=CARTESIAN_POINT('Origin',(-1.,-1.,35.640876193836));
#19826=CARTESIAN_POINT('',(-1.,-1.,35.640876193836));
#19827=CARTESIAN_POINT('',(-1.,-1.,35.7750503420619));
#19828=CARTESIAN_POINT('',(-1.,1.,35.640876193836));
#19829=CARTESIAN_POINT('',(-1.,1.,35.7750503420619));
#19830=CARTESIAN_POINT('',(-1.,-1.,35.640876193836));
#19831=CARTESIAN_POINT('Origin',(-1.45,-1.,35.4770895884162));
#19832=CARTESIAN_POINT('',(-1.45,-1.,35.4770895884162));
#19833=CARTESIAN_POINT('',(-1.,-1.,35.640876193836));
#19834=CARTESIAN_POINT('',(-1.45,1.,35.4770895884162));
#19835=CARTESIAN_POINT('',(-1.,1.,35.640876193836));
#19836=CARTESIAN_POINT('',(-1.45,-1.,35.4770895884162));
#19837=CARTESIAN_POINT('Origin',(-1.45,-1.,35.3105184167637));
#19838=CARTESIAN_POINT('',(-1.45,-1.,35.3105184167637));
#19839=CARTESIAN_POINT('',(-1.45,-1.,35.4770895884162));
#19840=CARTESIAN_POINT('',(-1.45,1.,35.3105184167637));
#19841=CARTESIAN_POINT('',(-1.45,1.,35.4770895884162));
#19842=CARTESIAN_POINT('',(-1.45,-1.,35.3105184167637));
#19843=CARTESIAN_POINT('Origin',(-1.,-1.,35.1467318113439));
#19844=CARTESIAN_POINT('',(-1.,-1.,35.1467318113439));
#19845=CARTESIAN_POINT('',(-1.45,-1.,35.3105184167637));
#19846=CARTESIAN_POINT('',(-1.,1.,35.1467318113439));
#19847=CARTESIAN_POINT('',(-1.45,1.,35.3105184167637));
#19848=CARTESIAN_POINT('',(-1.,-1.,35.1467318113439));
#19849=CARTESIAN_POINT('Origin',(-1.,-1.,35.0125576631181));
#19850=CARTESIAN_POINT('',(-1.,-1.,35.0125576631181));
#19851=CARTESIAN_POINT('',(-1.,-1.,35.1467318113439));
#19852=CARTESIAN_POINT('',(-1.,1.,35.0125576631181));
#19853=CARTESIAN_POINT('',(-1.,1.,35.1467318113439));
#19854=CARTESIAN_POINT('',(-1.,-1.,35.0125576631181));
#19855=CARTESIAN_POINT('Origin',(-1.45,-1.,34.8487710576983));
#19856=CARTESIAN_POINT('',(-1.45,-1.,34.8487710576983));
#19857=CARTESIAN_POINT('',(-1.,-1.,35.0125576631181));
#19858=CARTESIAN_POINT('',(-1.45,1.,34.8487710576983));
#19859=CARTESIAN_POINT('',(-1.,1.,35.0125576631181));
#19860=CARTESIAN_POINT('',(-1.45,-1.,34.8487710576983));
#19861=CARTESIAN_POINT('Origin',(-1.45,-1.,34.6821998860458));
#19862=CARTESIAN_POINT('',(-1.45,-1.,34.6821998860458));
#19863=CARTESIAN_POINT('',(-1.45,-1.,34.8487710576983));
#19864=CARTESIAN_POINT('',(-1.45,1.,34.6821998860458));
#19865=CARTESIAN_POINT('',(-1.45,1.,34.8487710576983));
#19866=CARTESIAN_POINT('',(-1.45,-1.,34.6821998860458));
#19867=CARTESIAN_POINT('Origin',(-1.,-1.,34.518413280626));
#19868=CARTESIAN_POINT('',(-1.,-1.,34.518413280626));
#19869=CARTESIAN_POINT('',(-1.45,-1.,34.6821998860458));
#19870=CARTESIAN_POINT('',(-1.,1.,34.518413280626));
#19871=CARTESIAN_POINT('',(-1.45,1.,34.6821998860458));
#19872=CARTESIAN_POINT('',(-1.,-1.,34.518413280626));
#19873=CARTESIAN_POINT('Origin',(-1.,-1.,34.3842391324001));
#19874=CARTESIAN_POINT('',(-1.,-1.,34.3842391324001));
#19875=CARTESIAN_POINT('',(-1.,-1.,34.518413280626));
#19876=CARTESIAN_POINT('',(-1.,1.,34.3842391324001));
#19877=CARTESIAN_POINT('',(-1.,1.,34.518413280626));
#19878=CARTESIAN_POINT('',(-1.,-1.,34.3842391324001));
#19879=CARTESIAN_POINT('Origin',(-1.45,-1.,34.2204525269803));
#19880=CARTESIAN_POINT('',(-1.45,-1.,34.2204525269803));
#19881=CARTESIAN_POINT('',(-1.,-1.,34.3842391324001));
#19882=CARTESIAN_POINT('',(-1.45,1.,34.2204525269803));
#19883=CARTESIAN_POINT('',(-1.,1.,34.3842391324001));
#19884=CARTESIAN_POINT('',(-1.45,-1.,34.2204525269803));
#19885=CARTESIAN_POINT('Origin',(-1.45,-1.,34.0538813553278));
#19886=CARTESIAN_POINT('',(-1.45,-1.,34.0538813553278));
#19887=CARTESIAN_POINT('',(-1.45,-1.,34.2204525269803));
#19888=CARTESIAN_POINT('',(-1.45,1.,34.0538813553278));
#19889=CARTESIAN_POINT('',(-1.45,1.,34.2204525269803));
#19890=CARTESIAN_POINT('',(-1.45,-1.,34.0538813553278));
#19891=CARTESIAN_POINT('Origin',(-1.,-1.,33.890094749908));
#19892=CARTESIAN_POINT('',(-1.,-1.,33.890094749908));
#19893=CARTESIAN_POINT('',(-1.45,-1.,34.0538813553278));
#19894=CARTESIAN_POINT('',(-1.,1.,33.890094749908));
#19895=CARTESIAN_POINT('',(-1.45,1.,34.0538813553278));
#19896=CARTESIAN_POINT('',(-1.,-1.,33.890094749908));
#19897=CARTESIAN_POINT('Origin',(-1.,-1.,33.7559206016821));
#19898=CARTESIAN_POINT('',(-1.,-1.,33.7559206016821));
#19899=CARTESIAN_POINT('',(-1.,-1.,33.890094749908));
#19900=CARTESIAN_POINT('',(-1.,1.,33.7559206016821));
#19901=CARTESIAN_POINT('',(-1.,1.,33.890094749908));
#19902=CARTESIAN_POINT('',(-1.,-1.,33.7559206016821));
#19903=CARTESIAN_POINT('Origin',(-1.45,-1.,33.5921339962624));
#19904=CARTESIAN_POINT('',(-1.45,-1.,33.5921339962624));
#19905=CARTESIAN_POINT('',(-1.,-1.,33.7559206016821));
#19906=CARTESIAN_POINT('',(-1.45,1.,33.5921339962624));
#19907=CARTESIAN_POINT('',(-1.,1.,33.7559206016821));
#19908=CARTESIAN_POINT('',(-1.45,-1.,33.5921339962624));
#19909=CARTESIAN_POINT('Origin',(-1.45,-1.,33.4255628246099));
#19910=CARTESIAN_POINT('',(-1.45,-1.,33.4255628246099));
#19911=CARTESIAN_POINT('',(-1.45,-1.,33.5921339962624));
#19912=CARTESIAN_POINT('',(-1.45,1.,33.4255628246099));
#19913=CARTESIAN_POINT('',(-1.45,1.,33.5921339962624));
#19914=CARTESIAN_POINT('',(-1.45,-1.,33.4255628246099));
#19915=CARTESIAN_POINT('Origin',(-1.,-1.,33.2617762191901));
#19916=CARTESIAN_POINT('',(-1.,-1.,33.2617762191901));
#19917=CARTESIAN_POINT('',(-1.45,-1.,33.4255628246099));
#19918=CARTESIAN_POINT('',(-1.,1.,33.2617762191901));
#19919=CARTESIAN_POINT('',(-1.45,1.,33.4255628246099));
#19920=CARTESIAN_POINT('',(-1.,-1.,33.2617762191901));
#19921=CARTESIAN_POINT('Origin',(-1.,-1.,33.1276020709642));
#19922=CARTESIAN_POINT('',(-1.,-1.,33.1276020709642));
#19923=CARTESIAN_POINT('',(-1.,-1.,33.2617762191901));
#19924=CARTESIAN_POINT('',(-1.,1.,33.1276020709642));
#19925=CARTESIAN_POINT('',(-1.,1.,33.2617762191901));
#19926=CARTESIAN_POINT('',(-1.,-1.,33.1276020709642));
#19927=CARTESIAN_POINT('Origin',(-1.45,-1.,32.9638154655444));
#19928=CARTESIAN_POINT('',(-1.45,-1.,32.9638154655444));
#19929=CARTESIAN_POINT('',(-1.,-1.,33.1276020709642));
#19930=CARTESIAN_POINT('',(-1.45,1.,32.9638154655444));
#19931=CARTESIAN_POINT('',(-1.,1.,33.1276020709642));
#19932=CARTESIAN_POINT('',(-1.45,-1.,32.9638154655444));
#19933=CARTESIAN_POINT('Origin',(-1.45,-1.,32.7972442938919));
#19934=CARTESIAN_POINT('',(-1.45,-1.,32.7972442938919));
#19935=CARTESIAN_POINT('',(-1.45,-1.,32.9638154655444));
#19936=CARTESIAN_POINT('',(-1.45,1.,32.7972442938919));
#19937=CARTESIAN_POINT('',(-1.45,1.,32.9638154655444));
#19938=CARTESIAN_POINT('',(-1.45,-1.,32.7972442938919));
#19939=CARTESIAN_POINT('Origin',(-1.,-1.,32.6334576884721));
#19940=CARTESIAN_POINT('',(-1.,-1.,32.6334576884721));
#19941=CARTESIAN_POINT('',(-1.45,-1.,32.7972442938919));
#19942=CARTESIAN_POINT('',(-1.,1.,32.6334576884721));
#19943=CARTESIAN_POINT('',(-1.45,1.,32.7972442938919));
#19944=CARTESIAN_POINT('',(-1.,-1.,32.6334576884721));
#19945=CARTESIAN_POINT('Origin',(-1.,-1.,32.4992835402462));
#19946=CARTESIAN_POINT('',(-1.,-1.,32.4992835402462));
#19947=CARTESIAN_POINT('',(-1.,-1.,32.6334576884721));
#19948=CARTESIAN_POINT('',(-1.,1.,32.4992835402462));
#19949=CARTESIAN_POINT('',(-1.,1.,32.6334576884721));
#19950=CARTESIAN_POINT('',(-1.,-1.,32.4992835402462));
#19951=CARTESIAN_POINT('Origin',(-1.45,-1.,32.3354969348264));
#19952=CARTESIAN_POINT('',(-1.45,-1.,32.3354969348264));
#19953=CARTESIAN_POINT('',(-1.,-1.,32.4992835402462));
#19954=CARTESIAN_POINT('',(-1.45,1.,32.3354969348264));
#19955=CARTESIAN_POINT('',(-1.,1.,32.4992835402462));
#19956=CARTESIAN_POINT('',(-1.45,-1.,32.3354969348264));
#19957=CARTESIAN_POINT('Origin',(-1.45,-1.,32.1689257631739));
#19958=CARTESIAN_POINT('',(-1.45,-1.,32.1689257631739));
#19959=CARTESIAN_POINT('',(-1.45,-1.,32.3354969348264));
#19960=CARTESIAN_POINT('',(-1.45,1.,32.1689257631739));
#19961=CARTESIAN_POINT('',(-1.45,1.,32.3354969348264));
#19962=CARTESIAN_POINT('',(-1.45,-1.,32.1689257631739));
#19963=CARTESIAN_POINT('Origin',(-1.,-1.,32.0051391577542));
#19964=CARTESIAN_POINT('',(-1.,-1.,32.0051391577542));
#19965=CARTESIAN_POINT('',(-1.45,-1.,32.1689257631739));
#19966=CARTESIAN_POINT('',(-1.,1.,32.0051391577542));
#19967=CARTESIAN_POINT('',(-1.45,1.,32.1689257631739));
#19968=CARTESIAN_POINT('',(-1.,-1.,32.0051391577542));
#19969=CARTESIAN_POINT('Origin',(-1.,-1.,31.8709650095283));
#19970=CARTESIAN_POINT('',(-1.,-1.,31.8709650095283));
#19971=CARTESIAN_POINT('',(-1.,-1.,32.0051391577542));
#19972=CARTESIAN_POINT('',(-1.,1.,31.8709650095283));
#19973=CARTESIAN_POINT('',(-1.,1.,32.0051391577542));
#19974=CARTESIAN_POINT('',(-1.,-1.,31.8709650095283));
#19975=CARTESIAN_POINT('Origin',(-1.45,-1.,31.7071784041085));
#19976=CARTESIAN_POINT('',(-1.45,-1.,31.7071784041085));
#19977=CARTESIAN_POINT('',(-1.,-1.,31.8709650095283));
#19978=CARTESIAN_POINT('',(-1.45,1.,31.7071784041085));
#19979=CARTESIAN_POINT('',(-1.,1.,31.8709650095283));
#19980=CARTESIAN_POINT('',(-1.45,-1.,31.7071784041085));
#19981=CARTESIAN_POINT('Origin',(-1.45,-1.,31.540607232456));
#19982=CARTESIAN_POINT('',(-1.45,-1.,31.540607232456));
#19983=CARTESIAN_POINT('',(-1.45,-1.,31.7071784041085));
#19984=CARTESIAN_POINT('',(-1.45,1.,31.540607232456));
#19985=CARTESIAN_POINT('',(-1.45,1.,31.7071784041085));
#19986=CARTESIAN_POINT('',(-1.45,-1.,31.540607232456));
#19987=CARTESIAN_POINT('Origin',(-1.,-1.,31.3768206270362));
#19988=CARTESIAN_POINT('',(-1.,-1.,31.3768206270362));
#19989=CARTESIAN_POINT('',(-1.45,-1.,31.540607232456));
#19990=CARTESIAN_POINT('',(-1.,1.,31.3768206270362));
#19991=CARTESIAN_POINT('',(-1.45,1.,31.540607232456));
#19992=CARTESIAN_POINT('',(-1.,-1.,31.3768206270362));
#19993=CARTESIAN_POINT('Origin',(-1.,-1.,31.2426464788103));
#19994=CARTESIAN_POINT('',(-1.,-1.,31.2426464788103));
#19995=CARTESIAN_POINT('',(-1.,-1.,31.3768206270362));
#19996=CARTESIAN_POINT('',(-1.,1.,31.2426464788103));
#19997=CARTESIAN_POINT('',(-1.,1.,31.3768206270362));
#19998=CARTESIAN_POINT('',(-1.,-1.,31.2426464788103));
#19999=CARTESIAN_POINT('Origin',(-1.45,-1.,31.0788598733905));
#20000=CARTESIAN_POINT('',(-1.45,-1.,31.0788598733905));
#20001=CARTESIAN_POINT('',(-1.,-1.,31.2426464788103));
#20002=CARTESIAN_POINT('',(-1.45,1.,31.0788598733905));
#20003=CARTESIAN_POINT('',(-1.,1.,31.2426464788103));
#20004=CARTESIAN_POINT('',(-1.45,-1.,31.0788598733905));
#20005=CARTESIAN_POINT('Origin',(-1.45,-1.,30.912288701738));
#20006=CARTESIAN_POINT('',(-1.45,-1.,30.912288701738));
#20007=CARTESIAN_POINT('',(-1.45,-1.,31.0788598733905));
#20008=CARTESIAN_POINT('',(-1.45,1.,30.912288701738));
#20009=CARTESIAN_POINT('',(-1.45,1.,31.0788598733905));
#20010=CARTESIAN_POINT('',(-1.45,-1.,30.912288701738));
#20011=CARTESIAN_POINT('Origin',(-1.,-1.,30.7485020963182));
#20012=CARTESIAN_POINT('',(-1.,-1.,30.7485020963182));
#20013=CARTESIAN_POINT('',(-1.45,-1.,30.912288701738));
#20014=CARTESIAN_POINT('',(-1.,1.,30.7485020963182));
#20015=CARTESIAN_POINT('',(-1.45,1.,30.912288701738));
#20016=CARTESIAN_POINT('',(-1.,-1.,30.7485020963182));
#20017=CARTESIAN_POINT('Origin',(-1.,-1.,30.6143279480924));
#20018=CARTESIAN_POINT('',(-1.,-1.,30.6143279480924));
#20019=CARTESIAN_POINT('',(-1.,-1.,30.7485020963182));
#20020=CARTESIAN_POINT('',(-1.,1.,30.6143279480924));
#20021=CARTESIAN_POINT('',(-1.,1.,30.7485020963182));
#20022=CARTESIAN_POINT('',(-1.,-1.,30.6143279480924));
#20023=CARTESIAN_POINT('Origin',(-1.45,-1.,30.4505413426726));
#20024=CARTESIAN_POINT('',(-1.45,-1.,30.4505413426726));
#20025=CARTESIAN_POINT('',(-1.,-1.,30.6143279480924));
#20026=CARTESIAN_POINT('',(-1.45,1.,30.4505413426726));
#20027=CARTESIAN_POINT('',(-1.,1.,30.6143279480924));
#20028=CARTESIAN_POINT('',(-1.45,-1.,30.4505413426726));
#20029=CARTESIAN_POINT('Origin',(-1.45,-1.,30.2839701710201));
#20030=CARTESIAN_POINT('',(-1.45,-1.,30.2839701710201));
#20031=CARTESIAN_POINT('',(-1.45,-1.,30.4505413426726));
#20032=CARTESIAN_POINT('',(-1.45,1.,30.2839701710201));
#20033=CARTESIAN_POINT('',(-1.45,1.,30.4505413426726));
#20034=CARTESIAN_POINT('',(-1.45,-1.,30.2839701710201));
#20035=CARTESIAN_POINT('Origin',(-1.,-1.,30.1201835656003));
#20036=CARTESIAN_POINT('',(-1.,-1.,30.1201835656003));
#20037=CARTESIAN_POINT('',(-1.45,-1.,30.2839701710201));
#20038=CARTESIAN_POINT('',(-1.,1.,30.1201835656003));
#20039=CARTESIAN_POINT('',(-1.45,1.,30.2839701710201));
#20040=CARTESIAN_POINT('',(-1.,-1.,30.1201835656003));
#20041=CARTESIAN_POINT('Origin',(-1.,-1.,29.9860094173744));
#20042=CARTESIAN_POINT('',(-1.,-1.,29.9860094173744));
#20043=CARTESIAN_POINT('',(-1.,-1.,30.1201835656003));
#20044=CARTESIAN_POINT('',(-1.,1.,29.9860094173744));
#20045=CARTESIAN_POINT('',(-1.,1.,30.1201835656003));
#20046=CARTESIAN_POINT('',(-1.,-1.,29.9860094173744));
#20047=CARTESIAN_POINT('Origin',(-1.45,-1.,29.8222228119546));
#20048=CARTESIAN_POINT('',(-1.45,-1.,29.8222228119546));
#20049=CARTESIAN_POINT('',(-1.,-1.,29.9860094173744));
#20050=CARTESIAN_POINT('',(-1.45,1.,29.8222228119546));
#20051=CARTESIAN_POINT('',(-1.,1.,29.9860094173744));
#20052=CARTESIAN_POINT('',(-1.45,-1.,29.8222228119546));
#20053=CARTESIAN_POINT('Origin',(-1.45,-1.,29.6556516403021));
#20054=CARTESIAN_POINT('',(-1.45,-1.,29.6556516403021));
#20055=CARTESIAN_POINT('',(-1.45,-1.,29.8222228119546));
#20056=CARTESIAN_POINT('',(-1.45,1.,29.6556516403021));
#20057=CARTESIAN_POINT('',(-1.45,1.,29.8222228119546));
#20058=CARTESIAN_POINT('',(-1.45,-1.,29.6556516403021));
#20059=CARTESIAN_POINT('Origin',(-1.,-1.,29.4918650348823));
#20060=CARTESIAN_POINT('',(-1.,-1.,29.4918650348823));
#20061=CARTESIAN_POINT('',(-1.45,-1.,29.6556516403021));
#20062=CARTESIAN_POINT('',(-1.,1.,29.4918650348823));
#20063=CARTESIAN_POINT('',(-1.45,1.,29.6556516403021));
#20064=CARTESIAN_POINT('',(-1.,-1.,29.4918650348823));
#20065=CARTESIAN_POINT('Origin',(-1.,-1.,29.3576908866564));
#20066=CARTESIAN_POINT('',(-1.,-1.,29.3576908866564));
#20067=CARTESIAN_POINT('',(-1.,-1.,29.4918650348823));
#20068=CARTESIAN_POINT('',(-1.,1.,29.3576908866564));
#20069=CARTESIAN_POINT('',(-1.,1.,29.4918650348823));
#20070=CARTESIAN_POINT('',(-1.,-1.,29.3576908866564));
#20071=CARTESIAN_POINT('Origin',(-1.45,-1.,29.1939042812366));
#20072=CARTESIAN_POINT('',(-1.45,-1.,29.1939042812366));
#20073=CARTESIAN_POINT('',(-1.,-1.,29.3576908866564));
#20074=CARTESIAN_POINT('',(-1.45,1.,29.1939042812366));
#20075=CARTESIAN_POINT('',(-1.,1.,29.3576908866564));
#20076=CARTESIAN_POINT('',(-1.45,-1.,29.1939042812366));
#20077=CARTESIAN_POINT('Origin',(-1.45,-1.,29.0273331095841));
#20078=CARTESIAN_POINT('',(-1.45,-1.,29.0273331095841));
#20079=CARTESIAN_POINT('',(-1.45,-1.,29.1939042812366));
#20080=CARTESIAN_POINT('',(-1.45,1.,29.0273331095841));
#20081=CARTESIAN_POINT('',(-1.45,1.,29.1939042812366));
#20082=CARTESIAN_POINT('',(-1.45,-1.,29.0273331095841));
#20083=CARTESIAN_POINT('Origin',(-1.,-1.,28.8635465041644));
#20084=CARTESIAN_POINT('',(-1.,-1.,28.8635465041644));
#20085=CARTESIAN_POINT('',(-1.45,-1.,29.0273331095841));
#20086=CARTESIAN_POINT('',(-1.,1.,28.8635465041644));
#20087=CARTESIAN_POINT('',(-1.45,1.,29.0273331095841));
#20088=CARTESIAN_POINT('',(-1.,-1.,28.8635465041644));
#20089=CARTESIAN_POINT('Origin',(-1.,-1.,28.7293723559385));
#20090=CARTESIAN_POINT('',(-1.,-1.,28.7293723559385));
#20091=CARTESIAN_POINT('',(-1.,-1.,28.8635465041644));
#20092=CARTESIAN_POINT('',(-1.,1.,28.7293723559385));
#20093=CARTESIAN_POINT('',(-1.,1.,28.8635465041644));
#20094=CARTESIAN_POINT('',(-1.,-1.,28.7293723559385));
#20095=CARTESIAN_POINT('Origin',(-1.45,-1.,28.5655857505187));
#20096=CARTESIAN_POINT('',(-1.45,-1.,28.5655857505187));
#20097=CARTESIAN_POINT('',(-1.,-1.,28.7293723559385));
#20098=CARTESIAN_POINT('',(-1.45,1.,28.5655857505187));
#20099=CARTESIAN_POINT('',(-1.,1.,28.7293723559385));
#20100=CARTESIAN_POINT('',(-1.45,-1.,28.5655857505187));
#20101=CARTESIAN_POINT('Origin',(-1.45,-1.,28.3990145788662));
#20102=CARTESIAN_POINT('',(-1.45,-1.,28.3990145788662));
#20103=CARTESIAN_POINT('',(-1.45,-1.,28.5655857505187));
#20104=CARTESIAN_POINT('',(-1.45,1.,28.3990145788662));
#20105=CARTESIAN_POINT('',(-1.45,1.,28.5655857505187));
#20106=CARTESIAN_POINT('',(-1.45,-1.,28.3990145788662));
#20107=CARTESIAN_POINT('Origin',(-1.,-1.,28.2352279734464));
#20108=CARTESIAN_POINT('',(-1.,-1.,28.2352279734464));
#20109=CARTESIAN_POINT('',(-1.45,-1.,28.3990145788662));
#20110=CARTESIAN_POINT('',(-1.,1.,28.2352279734464));
#20111=CARTESIAN_POINT('',(-1.45,1.,28.3990145788662));
#20112=CARTESIAN_POINT('',(-1.,-1.,28.2352279734464));
#20113=CARTESIAN_POINT('Origin',(-1.,-1.,28.1010538252205));
#20114=CARTESIAN_POINT('',(-1.,-1.,28.1010538252205));
#20115=CARTESIAN_POINT('',(-1.,-1.,28.2352279734464));
#20116=CARTESIAN_POINT('',(-1.,1.,28.1010538252205));
#20117=CARTESIAN_POINT('',(-1.,1.,28.2352279734464));
#20118=CARTESIAN_POINT('',(-1.,-1.,28.1010538252205));
#20119=CARTESIAN_POINT('Origin',(-1.45,-1.,27.9372672198007));
#20120=CARTESIAN_POINT('',(-1.45,-1.,27.9372672198007));
#20121=CARTESIAN_POINT('',(-1.,-1.,28.1010538252205));
#20122=CARTESIAN_POINT('',(-1.45,1.,27.9372672198007));
#20123=CARTESIAN_POINT('',(-1.,1.,28.1010538252205));
#20124=CARTESIAN_POINT('',(-1.45,-1.,27.9372672198007));
#20125=CARTESIAN_POINT('Origin',(-1.45,-1.,27.7706960481482));
#20126=CARTESIAN_POINT('',(-1.45,-1.,27.7706960481482));
#20127=CARTESIAN_POINT('',(-1.45,-1.,27.9372672198007));
#20128=CARTESIAN_POINT('',(-1.45,1.,27.7706960481482));
#20129=CARTESIAN_POINT('',(-1.45,1.,27.9372672198007));
#20130=CARTESIAN_POINT('',(-1.45,-1.,27.7706960481482));
#20131=CARTESIAN_POINT('Origin',(-1.,-1.,27.6069094427284));
#20132=CARTESIAN_POINT('',(-1.,-1.,27.6069094427284));
#20133=CARTESIAN_POINT('',(-1.45,-1.,27.7706960481482));
#20134=CARTESIAN_POINT('',(-1.,1.,27.6069094427284));
#20135=CARTESIAN_POINT('',(-1.45,1.,27.7706960481482));
#20136=CARTESIAN_POINT('',(-1.,-1.,27.6069094427284));
#20137=CARTESIAN_POINT('Origin',(-1.,-1.,27.4727352945026));
#20138=CARTESIAN_POINT('',(-1.,-1.,27.4727352945026));
#20139=CARTESIAN_POINT('',(-1.,-1.,27.6069094427284));
#20140=CARTESIAN_POINT('',(-1.,1.,27.4727352945026));
#20141=CARTESIAN_POINT('',(-1.,1.,27.6069094427284));
#20142=CARTESIAN_POINT('',(-1.,-1.,27.4727352945026));
#20143=CARTESIAN_POINT('Origin',(-1.45,-1.,27.3089486890828));
#20144=CARTESIAN_POINT('',(-1.45,-1.,27.3089486890828));
#20145=CARTESIAN_POINT('',(-1.,-1.,27.4727352945026));
#20146=CARTESIAN_POINT('',(-1.45,1.,27.3089486890828));
#20147=CARTESIAN_POINT('',(-1.,1.,27.4727352945026));
#20148=CARTESIAN_POINT('',(-1.45,-1.,27.3089486890828));
#20149=CARTESIAN_POINT('Origin',(-1.45,-1.,27.1423775174303));
#20150=CARTESIAN_POINT('',(-1.45,-1.,27.1423775174303));
#20151=CARTESIAN_POINT('',(-1.45,-1.,27.3089486890828));
#20152=CARTESIAN_POINT('',(-1.45,1.,27.1423775174303));
#20153=CARTESIAN_POINT('',(-1.45,1.,27.3089486890828));
#20154=CARTESIAN_POINT('',(-1.45,-1.,27.1423775174303));
#20155=CARTESIAN_POINT('Origin',(-1.,-1.,26.9785909120105));
#20156=CARTESIAN_POINT('',(-1.,-1.,26.9785909120105));
#20157=CARTESIAN_POINT('',(-1.45,-1.,27.1423775174303));
#20158=CARTESIAN_POINT('',(-1.,1.,26.9785909120105));
#20159=CARTESIAN_POINT('',(-1.45,1.,27.1423775174303));
#20160=CARTESIAN_POINT('',(-1.,-1.,26.9785909120105));
#20161=CARTESIAN_POINT('Origin',(-1.,-1.,26.8444167637846));
#20162=CARTESIAN_POINT('',(-1.,-1.,26.8444167637846));
#20163=CARTESIAN_POINT('',(-1.,-1.,26.9785909120105));
#20164=CARTESIAN_POINT('',(-1.,1.,26.8444167637846));
#20165=CARTESIAN_POINT('',(-1.,1.,26.9785909120105));
#20166=CARTESIAN_POINT('',(-1.,-1.,26.8444167637846));
#20167=CARTESIAN_POINT('Origin',(-1.45,-1.,26.6806301583648));
#20168=CARTESIAN_POINT('',(-1.45,-1.,26.6806301583648));
#20169=CARTESIAN_POINT('',(-1.,-1.,26.8444167637846));
#20170=CARTESIAN_POINT('',(-1.45,1.,26.6806301583648));
#20171=CARTESIAN_POINT('',(-1.,1.,26.8444167637846));
#20172=CARTESIAN_POINT('',(-1.45,-1.,26.6806301583648));
#20173=CARTESIAN_POINT('Origin',(-1.45,-1.,26.5140589867123));
#20174=CARTESIAN_POINT('',(-1.45,-1.,26.5140589867123));
#20175=CARTESIAN_POINT('',(-1.45,-1.,26.6806301583648));
#20176=CARTESIAN_POINT('',(-1.45,1.,26.5140589867123));
#20177=CARTESIAN_POINT('',(-1.45,1.,26.6806301583648));
#20178=CARTESIAN_POINT('',(-1.45,-1.,26.5140589867123));
#20179=CARTESIAN_POINT('Origin',(-1.,-1.,26.3502723812925));
#20180=CARTESIAN_POINT('',(-1.,-1.,26.3502723812925));
#20181=CARTESIAN_POINT('',(-1.45,-1.,26.5140589867123));
#20182=CARTESIAN_POINT('',(-1.,1.,26.3502723812925));
#20183=CARTESIAN_POINT('',(-1.45,1.,26.5140589867123));
#20184=CARTESIAN_POINT('',(-1.,-1.,26.3502723812925));
#20185=CARTESIAN_POINT('Origin',(-1.,-1.,26.2160982330666));
#20186=CARTESIAN_POINT('',(-1.,-1.,26.2160982330666));
#20187=CARTESIAN_POINT('',(-1.,-1.,26.3502723812925));
#20188=CARTESIAN_POINT('',(-1.,1.,26.2160982330666));
#20189=CARTESIAN_POINT('',(-1.,1.,26.3502723812925));
#20190=CARTESIAN_POINT('',(-1.,-1.,26.2160982330666));
#20191=CARTESIAN_POINT('Origin',(-1.45,-1.,26.0523116276469));
#20192=CARTESIAN_POINT('',(-1.45,-1.,26.0523116276469));
#20193=CARTESIAN_POINT('',(-1.,-1.,26.2160982330666));
#20194=CARTESIAN_POINT('',(-1.45,1.,26.0523116276469));
#20195=CARTESIAN_POINT('',(-1.,1.,26.2160982330666));
#20196=CARTESIAN_POINT('',(-1.45,-1.,26.0523116276469));
#20197=CARTESIAN_POINT('Origin',(-1.45,-1.,25.8857404559944));
#20198=CARTESIAN_POINT('',(-1.45,-1.,25.8857404559944));
#20199=CARTESIAN_POINT('',(-1.45,-1.,26.0523116276469));
#20200=CARTESIAN_POINT('',(-1.45,1.,25.8857404559944));
#20201=CARTESIAN_POINT('',(-1.45,1.,26.0523116276469));
#20202=CARTESIAN_POINT('',(-1.45,-1.,25.8857404559944));
#20203=CARTESIAN_POINT('Origin',(-1.,-1.,25.7219538505746));
#20204=CARTESIAN_POINT('',(-1.,-1.,25.7219538505746));
#20205=CARTESIAN_POINT('',(-1.45,-1.,25.8857404559944));
#20206=CARTESIAN_POINT('',(-1.,1.,25.7219538505746));
#20207=CARTESIAN_POINT('',(-1.45,1.,25.8857404559944));
#20208=CARTESIAN_POINT('',(-1.,-1.,25.7219538505746));
#20209=CARTESIAN_POINT('Origin',(-1.,-1.,25.5877797023487));
#20210=CARTESIAN_POINT('',(-1.,-1.,25.5877797023487));
#20211=CARTESIAN_POINT('',(-1.,-1.,25.7219538505746));
#20212=CARTESIAN_POINT('',(-1.,1.,25.5877797023487));
#20213=CARTESIAN_POINT('',(-1.,1.,25.7219538505746));
#20214=CARTESIAN_POINT('',(-1.,-1.,25.5877797023487));
#20215=CARTESIAN_POINT('Origin',(-1.45,-1.,25.4239930969289));
#20216=CARTESIAN_POINT('',(-1.45,-1.,25.4239930969289));
#20217=CARTESIAN_POINT('',(-1.,-1.,25.5877797023487));
#20218=CARTESIAN_POINT('',(-1.45,1.,25.4239930969289));
#20219=CARTESIAN_POINT('',(-1.,1.,25.5877797023487));
#20220=CARTESIAN_POINT('',(-1.45,-1.,25.4239930969289));
#20221=CARTESIAN_POINT('Origin',(-1.45,-1.,25.2574219252764));
#20222=CARTESIAN_POINT('',(-1.45,-1.,25.2574219252764));
#20223=CARTESIAN_POINT('',(-1.45,-1.,25.4239930969289));
#20224=CARTESIAN_POINT('',(-1.45,1.,25.2574219252764));
#20225=CARTESIAN_POINT('',(-1.45,1.,25.4239930969289));
#20226=CARTESIAN_POINT('',(-1.45,-1.,25.2574219252764));
#20227=CARTESIAN_POINT('Origin',(-1.,-1.,25.0936353198566));
#20228=CARTESIAN_POINT('',(-1.,-1.,25.0936353198566));
#20229=CARTESIAN_POINT('',(-1.45,-1.,25.2574219252764));
#20230=CARTESIAN_POINT('',(-1.,1.,25.0936353198566));
#20231=CARTESIAN_POINT('',(-1.45,1.,25.2574219252764));
#20232=CARTESIAN_POINT('',(-1.,-1.,25.0936353198566));
#20233=CARTESIAN_POINT('Origin',(-1.,-1.,24.9594611716307));
#20234=CARTESIAN_POINT('',(-1.,-1.,24.9594611716307));
#20235=CARTESIAN_POINT('',(-1.,-1.,25.0936353198566));
#20236=CARTESIAN_POINT('',(-1.,1.,24.9594611716307));
#20237=CARTESIAN_POINT('',(-1.,1.,25.0936353198566));
#20238=CARTESIAN_POINT('',(-1.,-1.,24.9594611716307));
#20239=CARTESIAN_POINT('Origin',(-1.45,-1.,24.7956745662109));
#20240=CARTESIAN_POINT('',(-1.45,-1.,24.7956745662109));
#20241=CARTESIAN_POINT('',(-1.,-1.,24.9594611716307));
#20242=CARTESIAN_POINT('',(-1.45,1.,24.7956745662109));
#20243=CARTESIAN_POINT('',(-1.,1.,24.9594611716307));
#20244=CARTESIAN_POINT('',(-1.45,-1.,24.7956745662109));
#20245=CARTESIAN_POINT('Origin',(-1.45,-1.,24.6291033945584));
#20246=CARTESIAN_POINT('',(-1.45,-1.,24.6291033945584));
#20247=CARTESIAN_POINT('',(-1.45,-1.,24.7956745662109));
#20248=CARTESIAN_POINT('',(-1.45,1.,24.6291033945584));
#20249=CARTESIAN_POINT('',(-1.45,1.,24.7956745662109));
#20250=CARTESIAN_POINT('',(-1.45,-1.,24.6291033945584));
#20251=CARTESIAN_POINT('Origin',(-1.,-1.,24.4653167891386));
#20252=CARTESIAN_POINT('',(-1.,-1.,24.4653167891386));
#20253=CARTESIAN_POINT('',(-1.45,-1.,24.6291033945584));
#20254=CARTESIAN_POINT('',(-1.,1.,24.4653167891386));
#20255=CARTESIAN_POINT('',(-1.45,1.,24.6291033945584));
#20256=CARTESIAN_POINT('',(-1.,-1.,24.4653167891386));
#20257=CARTESIAN_POINT('Origin',(-1.,-1.,24.3311426409128));
#20258=CARTESIAN_POINT('',(-1.,-1.,24.3311426409128));
#20259=CARTESIAN_POINT('',(-1.,-1.,24.4653167891386));
#20260=CARTESIAN_POINT('',(-1.,1.,24.3311426409128));
#20261=CARTESIAN_POINT('',(-1.,1.,24.4653167891386));
#20262=CARTESIAN_POINT('',(-1.,-1.,24.3311426409128));
#20263=CARTESIAN_POINT('Origin',(-1.45,-1.,24.167356035493));
#20264=CARTESIAN_POINT('',(-1.45,-1.,24.167356035493));
#20265=CARTESIAN_POINT('',(-1.,-1.,24.3311426409128));
#20266=CARTESIAN_POINT('',(-1.45,1.,24.167356035493));
#20267=CARTESIAN_POINT('',(-1.,1.,24.3311426409128));
#20268=CARTESIAN_POINT('',(-1.45,-1.,24.167356035493));
#20269=CARTESIAN_POINT('Origin',(-1.45,-1.,24.0007848638405));
#20270=CARTESIAN_POINT('',(-1.45,-1.,24.0007848638405));
#20271=CARTESIAN_POINT('',(-1.45,-1.,24.167356035493));
#20272=CARTESIAN_POINT('',(-1.45,1.,24.0007848638405));
#20273=CARTESIAN_POINT('',(-1.45,1.,24.167356035493));
#20274=CARTESIAN_POINT('',(-1.45,-1.,24.0007848638405));
#20275=CARTESIAN_POINT('Origin',(-1.,-1.,23.8369982584207));
#20276=CARTESIAN_POINT('',(-1.,-1.,23.8369982584207));
#20277=CARTESIAN_POINT('',(-1.45,-1.,24.0007848638405));
#20278=CARTESIAN_POINT('',(-1.,1.,23.8369982584207));
#20279=CARTESIAN_POINT('',(-1.45,1.,24.0007848638405));
#20280=CARTESIAN_POINT('',(-1.,-1.,23.8369982584207));
#20281=CARTESIAN_POINT('Origin',(-1.,-1.,23.7028241101948));
#20282=CARTESIAN_POINT('',(-1.,-1.,23.7028241101948));
#20283=CARTESIAN_POINT('',(-1.,-1.,23.8369982584207));
#20284=CARTESIAN_POINT('',(-1.,1.,23.7028241101948));
#20285=CARTESIAN_POINT('',(-1.,1.,23.8369982584207));
#20286=CARTESIAN_POINT('',(-1.,-1.,23.7028241101948));
#20287=CARTESIAN_POINT('Origin',(-1.45,-1.,23.539037504775));
#20288=CARTESIAN_POINT('',(-1.45,-1.,23.539037504775));
#20289=CARTESIAN_POINT('',(-1.,-1.,23.7028241101948));
#20290=CARTESIAN_POINT('',(-1.45,1.,23.539037504775));
#20291=CARTESIAN_POINT('',(-1.,1.,23.7028241101948));
#20292=CARTESIAN_POINT('',(-1.45,-1.,23.539037504775));
#20293=CARTESIAN_POINT('Origin',(-1.45,-1.,23.3724663331225));
#20294=CARTESIAN_POINT('',(-1.45,-1.,23.3724663331225));
#20295=CARTESIAN_POINT('',(-1.45,-1.,23.539037504775));
#20296=CARTESIAN_POINT('',(-1.45,1.,23.3724663331225));
#20297=CARTESIAN_POINT('',(-1.45,1.,23.539037504775));
#20298=CARTESIAN_POINT('',(-1.45,-1.,23.3724663331225));
#20299=CARTESIAN_POINT('Origin',(-1.,-1.,23.2086797277027));
#20300=CARTESIAN_POINT('',(-1.,-1.,23.2086797277027));
#20301=CARTESIAN_POINT('',(-1.45,-1.,23.3724663331225));
#20302=CARTESIAN_POINT('',(-1.,1.,23.2086797277027));
#20303=CARTESIAN_POINT('',(-1.45,1.,23.3724663331225));
#20304=CARTESIAN_POINT('',(-1.,-1.,23.2086797277027));
#20305=CARTESIAN_POINT('Origin',(-1.,-1.,23.0745055794769));
#20306=CARTESIAN_POINT('',(-1.,-1.,23.0745055794769));
#20307=CARTESIAN_POINT('',(-1.,-1.,23.2086797277027));
#20308=CARTESIAN_POINT('',(-1.,1.,23.0745055794769));
#20309=CARTESIAN_POINT('',(-1.,1.,23.2086797277027));
#20310=CARTESIAN_POINT('',(-1.,-1.,23.0745055794769));
#20311=CARTESIAN_POINT('Origin',(-1.45,-1.,22.9107189740571));
#20312=CARTESIAN_POINT('',(-1.45,-1.,22.9107189740571));
#20313=CARTESIAN_POINT('',(-1.,-1.,23.0745055794769));
#20314=CARTESIAN_POINT('',(-1.45,1.,22.9107189740571));
#20315=CARTESIAN_POINT('',(-1.,1.,23.0745055794769));
#20316=CARTESIAN_POINT('',(-1.45,-1.,22.9107189740571));
#20317=CARTESIAN_POINT('Origin',(-1.45,-1.,22.7441478024046));
#20318=CARTESIAN_POINT('',(-1.45,-1.,22.7441478024046));
#20319=CARTESIAN_POINT('',(-1.45,-1.,22.9107189740571));
#20320=CARTESIAN_POINT('',(-1.45,1.,22.7441478024046));
#20321=CARTESIAN_POINT('',(-1.45,1.,22.9107189740571));
#20322=CARTESIAN_POINT('',(-1.45,-1.,22.7441478024046));
#20323=CARTESIAN_POINT('Origin',(-1.,-1.,22.5803611969848));
#20324=CARTESIAN_POINT('',(-1.,-1.,22.5803611969848));
#20325=CARTESIAN_POINT('',(-1.45,-1.,22.7441478024046));
#20326=CARTESIAN_POINT('',(-1.,1.,22.5803611969848));
#20327=CARTESIAN_POINT('',(-1.45,1.,22.7441478024046));
#20328=CARTESIAN_POINT('',(-1.,-1.,22.5803611969848));
#20329=CARTESIAN_POINT('Origin',(-1.,-1.,22.4461870487589));
#20330=CARTESIAN_POINT('',(-1.,-1.,22.4461870487589));
#20331=CARTESIAN_POINT('',(-1.,-1.,22.5803611969848));
#20332=CARTESIAN_POINT('',(-1.,1.,22.4461870487589));
#20333=CARTESIAN_POINT('',(-1.,1.,22.5803611969848));
#20334=CARTESIAN_POINT('',(-1.,-1.,22.4461870487589));
#20335=CARTESIAN_POINT('Origin',(-1.45,-1.,22.2824004433391));
#20336=CARTESIAN_POINT('',(-1.45,-1.,22.2824004433391));
#20337=CARTESIAN_POINT('',(-1.,-1.,22.4461870487589));
#20338=CARTESIAN_POINT('',(-1.45,1.,22.2824004433391));
#20339=CARTESIAN_POINT('',(-1.,1.,22.4461870487589));
#20340=CARTESIAN_POINT('',(-1.45,-1.,22.2824004433391));
#20341=CARTESIAN_POINT('Origin',(-1.45,-1.,22.1158292716866));
#20342=CARTESIAN_POINT('',(-1.45,-1.,22.1158292716866));
#20343=CARTESIAN_POINT('',(-1.45,-1.,22.2824004433391));
#20344=CARTESIAN_POINT('',(-1.45,1.,22.1158292716866));
#20345=CARTESIAN_POINT('',(-1.45,1.,22.2824004433391));
#20346=CARTESIAN_POINT('',(-1.45,-1.,22.1158292716866));
#20347=CARTESIAN_POINT('Origin',(-1.,-1.,21.9520426662668));
#20348=CARTESIAN_POINT('',(-1.,-1.,21.9520426662668));
#20349=CARTESIAN_POINT('',(-1.45,-1.,22.1158292716866));
#20350=CARTESIAN_POINT('',(-1.,1.,21.9520426662668));
#20351=CARTESIAN_POINT('',(-1.45,1.,22.1158292716866));
#20352=CARTESIAN_POINT('',(-1.,-1.,21.9520426662668));
#20353=CARTESIAN_POINT('Origin',(-1.,-1.,21.8178685180409));
#20354=CARTESIAN_POINT('',(-1.,-1.,21.8178685180409));
#20355=CARTESIAN_POINT('',(-1.,-1.,21.9520426662668));
#20356=CARTESIAN_POINT('',(-1.,1.,21.8178685180409));
#20357=CARTESIAN_POINT('',(-1.,1.,21.9520426662668));
#20358=CARTESIAN_POINT('',(-1.,-1.,21.8178685180409));
#20359=CARTESIAN_POINT('Origin',(-1.45,-1.,21.6540819126211));
#20360=CARTESIAN_POINT('',(-1.45,-1.,21.6540819126211));
#20361=CARTESIAN_POINT('',(-1.,-1.,21.8178685180409));
#20362=CARTESIAN_POINT('',(-1.45,1.,21.6540819126211));
#20363=CARTESIAN_POINT('',(-1.,1.,21.8178685180409));
#20364=CARTESIAN_POINT('',(-1.45,-1.,21.6540819126211));
#20365=CARTESIAN_POINT('Origin',(-1.45,-1.,21.4875107409686));
#20366=CARTESIAN_POINT('',(-1.45,-1.,21.4875107409686));
#20367=CARTESIAN_POINT('',(-1.45,-1.,21.6540819126211));
#20368=CARTESIAN_POINT('',(-1.45,1.,21.4875107409686));
#20369=CARTESIAN_POINT('',(-1.45,1.,21.6540819126211));
#20370=CARTESIAN_POINT('',(-1.45,-1.,21.4875107409686));
#20371=CARTESIAN_POINT('Origin',(-1.,-1.,21.3237241355489));
#20372=CARTESIAN_POINT('',(-1.,-1.,21.3237241355489));
#20373=CARTESIAN_POINT('',(-1.45,-1.,21.4875107409686));
#20374=CARTESIAN_POINT('',(-1.,1.,21.3237241355489));
#20375=CARTESIAN_POINT('',(-1.45,1.,21.4875107409686));
#20376=CARTESIAN_POINT('',(-1.,-1.,21.3237241355489));
#20377=CARTESIAN_POINT('Origin',(-1.,-1.,21.189549987323));
#20378=CARTESIAN_POINT('',(-1.,-1.,21.189549987323));
#20379=CARTESIAN_POINT('',(-1.,-1.,21.3237241355489));
#20380=CARTESIAN_POINT('',(-1.,1.,21.189549987323));
#20381=CARTESIAN_POINT('',(-1.,1.,21.3237241355489));
#20382=CARTESIAN_POINT('',(-1.,-1.,21.189549987323));
#20383=CARTESIAN_POINT('Origin',(-1.45,-1.,21.0257633819032));
#20384=CARTESIAN_POINT('',(-1.45,-1.,21.0257633819032));
#20385=CARTESIAN_POINT('',(-1.,-1.,21.189549987323));
#20386=CARTESIAN_POINT('',(-1.45,1.,21.0257633819032));
#20387=CARTESIAN_POINT('',(-1.,1.,21.189549987323));
#20388=CARTESIAN_POINT('',(-1.45,-1.,21.0257633819032));
#20389=CARTESIAN_POINT('Origin',(-1.45,-1.,20.8591922102507));
#20390=CARTESIAN_POINT('',(-1.45,-1.,20.8591922102507));
#20391=CARTESIAN_POINT('',(-1.45,-1.,21.0257633819032));
#20392=CARTESIAN_POINT('',(-1.45,1.,20.8591922102507));
#20393=CARTESIAN_POINT('',(-1.45,1.,21.0257633819032));
#20394=CARTESIAN_POINT('',(-1.45,-1.,20.8591922102507));
#20395=CARTESIAN_POINT('Origin',(-1.,-1.,20.6954056048309));
#20396=CARTESIAN_POINT('',(-1.,-1.,20.6954056048309));
#20397=CARTESIAN_POINT('',(-1.45,-1.,20.8591922102507));
#20398=CARTESIAN_POINT('',(-1.,1.,20.6954056048309));
#20399=CARTESIAN_POINT('',(-1.45,1.,20.8591922102507));
#20400=CARTESIAN_POINT('',(-1.,-1.,20.6954056048309));
#20401=CARTESIAN_POINT('Origin',(-1.,-1.,20.561231456605));
#20402=CARTESIAN_POINT('',(-1.,-1.,20.561231456605));
#20403=CARTESIAN_POINT('',(-1.,-1.,20.6954056048309));
#20404=CARTESIAN_POINT('',(-1.,1.,20.561231456605));
#20405=CARTESIAN_POINT('',(-1.,1.,20.6954056048309));
#20406=CARTESIAN_POINT('',(-1.,-1.,20.561231456605));
#20407=CARTESIAN_POINT('Origin',(-1.45,-1.,20.3974448511852));
#20408=CARTESIAN_POINT('',(-1.45,-1.,20.3974448511852));
#20409=CARTESIAN_POINT('',(-1.,-1.,20.561231456605));
#20410=CARTESIAN_POINT('',(-1.45,1.,20.3974448511852));
#20411=CARTESIAN_POINT('',(-1.,1.,20.561231456605));
#20412=CARTESIAN_POINT('',(-1.45,-1.,20.3974448511852));
#20413=CARTESIAN_POINT('Origin',(-1.45,-1.,20.2308736795327));
#20414=CARTESIAN_POINT('',(-1.45,-1.,20.2308736795327));
#20415=CARTESIAN_POINT('',(-1.45,-1.,20.3974448511852));
#20416=CARTESIAN_POINT('',(-1.45,1.,20.2308736795327));
#20417=CARTESIAN_POINT('',(-1.45,1.,20.3974448511852));
#20418=CARTESIAN_POINT('',(-1.45,-1.,20.2308736795327));
#20419=CARTESIAN_POINT('Origin',(-1.,-1.,20.0670870741129));
#20420=CARTESIAN_POINT('',(-1.,-1.,20.0670870741129));
#20421=CARTESIAN_POINT('',(-1.45,-1.,20.2308736795327));
#20422=CARTESIAN_POINT('',(-1.,1.,20.0670870741129));
#20423=CARTESIAN_POINT('',(-1.45,1.,20.2308736795327));
#20424=CARTESIAN_POINT('',(-1.,-1.,20.0670870741129));
#20425=CARTESIAN_POINT('Origin',(-1.,-1.,19.9329129258871));
#20426=CARTESIAN_POINT('',(-1.,-1.,19.9329129258871));
#20427=CARTESIAN_POINT('',(-1.,-1.,20.0670870741129));
#20428=CARTESIAN_POINT('',(-1.,1.,19.9329129258871));
#20429=CARTESIAN_POINT('',(-1.,1.,20.0670870741129));
#20430=CARTESIAN_POINT('',(-1.,-1.,19.9329129258871));
#20431=CARTESIAN_POINT('Origin',(-1.45,-1.,19.7691263204673));
#20432=CARTESIAN_POINT('',(-1.45,-1.,19.7691263204673));
#20433=CARTESIAN_POINT('',(-1.,-1.,19.9329129258871));
#20434=CARTESIAN_POINT('',(-1.45,1.,19.7691263204673));
#20435=CARTESIAN_POINT('',(-1.,1.,19.9329129258871));
#20436=CARTESIAN_POINT('',(-1.45,-1.,19.7691263204673));
#20437=CARTESIAN_POINT('Origin',(-1.45,-1.,19.6025551488148));
#20438=CARTESIAN_POINT('',(-1.45,-1.,19.6025551488148));
#20439=CARTESIAN_POINT('',(-1.45,-1.,19.7691263204673));
#20440=CARTESIAN_POINT('',(-1.45,1.,19.6025551488148));
#20441=CARTESIAN_POINT('',(-1.45,1.,19.7691263204673));
#20442=CARTESIAN_POINT('',(-1.45,-1.,19.6025551488148));
#20443=CARTESIAN_POINT('Origin',(-1.,-1.,19.438768543395));
#20444=CARTESIAN_POINT('',(-1.,-1.,19.438768543395));
#20445=CARTESIAN_POINT('',(-1.45,-1.,19.6025551488148));
#20446=CARTESIAN_POINT('',(-1.,1.,19.438768543395));
#20447=CARTESIAN_POINT('',(-1.45,1.,19.6025551488148));
#20448=CARTESIAN_POINT('',(-1.,-1.,19.438768543395));
#20449=CARTESIAN_POINT('Origin',(-1.,-1.,19.3045943951691));
#20450=CARTESIAN_POINT('',(-1.,-1.,19.3045943951691));
#20451=CARTESIAN_POINT('',(-1.,-1.,19.438768543395));
#20452=CARTESIAN_POINT('',(-1.,1.,19.3045943951691));
#20453=CARTESIAN_POINT('',(-1.,1.,19.438768543395));
#20454=CARTESIAN_POINT('',(-1.,-1.,19.3045943951691));
#20455=CARTESIAN_POINT('Origin',(-1.45,-1.,19.1408077897493));
#20456=CARTESIAN_POINT('',(-1.45,-1.,19.1408077897493));
#20457=CARTESIAN_POINT('',(-1.,-1.,19.3045943951691));
#20458=CARTESIAN_POINT('',(-1.45,1.,19.1408077897493));
#20459=CARTESIAN_POINT('',(-1.,1.,19.3045943951691));
#20460=CARTESIAN_POINT('',(-1.45,-1.,19.1408077897493));
#20461=CARTESIAN_POINT('Origin',(-1.45,-1.,18.9742366180968));
#20462=CARTESIAN_POINT('',(-1.45,-1.,18.9742366180968));
#20463=CARTESIAN_POINT('',(-1.45,-1.,19.1408077897493));
#20464=CARTESIAN_POINT('',(-1.45,1.,18.9742366180968));
#20465=CARTESIAN_POINT('',(-1.45,1.,19.1408077897493));
#20466=CARTESIAN_POINT('',(-1.45,-1.,18.9742366180968));
#20467=CARTESIAN_POINT('Origin',(-1.,-1.,18.810450012677));
#20468=CARTESIAN_POINT('',(-1.,-1.,18.810450012677));
#20469=CARTESIAN_POINT('',(-1.45,-1.,18.9742366180968));
#20470=CARTESIAN_POINT('',(-1.,1.,18.810450012677));
#20471=CARTESIAN_POINT('',(-1.45,1.,18.9742366180968));
#20472=CARTESIAN_POINT('',(-1.,-1.,18.810450012677));
#20473=CARTESIAN_POINT('Origin',(-1.,-1.,18.6762758644511));
#20474=CARTESIAN_POINT('',(-1.,-1.,18.6762758644511));
#20475=CARTESIAN_POINT('',(-1.,-1.,18.810450012677));
#20476=CARTESIAN_POINT('',(-1.,1.,18.6762758644511));
#20477=CARTESIAN_POINT('',(-1.,1.,18.810450012677));
#20478=CARTESIAN_POINT('',(-1.,-1.,18.6762758644511));
#20479=CARTESIAN_POINT('Origin',(-1.45,-1.,18.5124892590314));
#20480=CARTESIAN_POINT('',(-1.45,-1.,18.5124892590314));
#20481=CARTESIAN_POINT('',(-1.,-1.,18.6762758644511));
#20482=CARTESIAN_POINT('',(-1.45,1.,18.5124892590314));
#20483=CARTESIAN_POINT('',(-1.,1.,18.6762758644511));
#20484=CARTESIAN_POINT('',(-1.45,-1.,18.5124892590314));
#20485=CARTESIAN_POINT('Origin',(-1.45,-1.,18.3459180873789));
#20486=CARTESIAN_POINT('',(-1.45,-1.,18.3459180873789));
#20487=CARTESIAN_POINT('',(-1.45,-1.,18.5124892590314));
#20488=CARTESIAN_POINT('',(-1.45,1.,18.3459180873789));
#20489=CARTESIAN_POINT('',(-1.45,1.,18.5124892590314));
#20490=CARTESIAN_POINT('',(-1.45,-1.,18.3459180873789));
#20491=CARTESIAN_POINT('Origin',(-1.,-1.,18.1821314819591));
#20492=CARTESIAN_POINT('',(-1.,-1.,18.1821314819591));
#20493=CARTESIAN_POINT('',(-1.45,-1.,18.3459180873789));
#20494=CARTESIAN_POINT('',(-1.,1.,18.1821314819591));
#20495=CARTESIAN_POINT('',(-1.45,1.,18.3459180873789));
#20496=CARTESIAN_POINT('',(-1.,-1.,18.1821314819591));
#20497=CARTESIAN_POINT('Origin',(-1.,-1.,18.0479573337332));
#20498=CARTESIAN_POINT('',(-1.,-1.,18.0479573337332));
#20499=CARTESIAN_POINT('',(-1.,-1.,18.1821314819591));
#20500=CARTESIAN_POINT('',(-1.,1.,18.0479573337332));
#20501=CARTESIAN_POINT('',(-1.,1.,18.1821314819591));
#20502=CARTESIAN_POINT('',(-1.,-1.,18.0479573337332));
#20503=CARTESIAN_POINT('Origin',(-1.45,-1.,17.8841707283134));
#20504=CARTESIAN_POINT('',(-1.45,-1.,17.8841707283134));
#20505=CARTESIAN_POINT('',(-1.,-1.,18.0479573337332));
#20506=CARTESIAN_POINT('',(-1.45,1.,17.8841707283134));
#20507=CARTESIAN_POINT('',(-1.,1.,18.0479573337332));
#20508=CARTESIAN_POINT('',(-1.45,-1.,17.8841707283134));
#20509=CARTESIAN_POINT('Origin',(-1.45,-1.,17.7175995566609));
#20510=CARTESIAN_POINT('',(-1.45,-1.,17.7175995566609));
#20511=CARTESIAN_POINT('',(-1.45,-1.,17.8841707283134));
#20512=CARTESIAN_POINT('',(-1.45,1.,17.7175995566609));
#20513=CARTESIAN_POINT('',(-1.45,1.,17.8841707283134));
#20514=CARTESIAN_POINT('',(-1.45,-1.,17.7175995566609));
#20515=CARTESIAN_POINT('Origin',(-1.,-1.,17.5538129512411));
#20516=CARTESIAN_POINT('',(-1.,-1.,17.5538129512411));
#20517=CARTESIAN_POINT('',(-1.45,-1.,17.7175995566609));
#20518=CARTESIAN_POINT('',(-1.,1.,17.5538129512411));
#20519=CARTESIAN_POINT('',(-1.45,1.,17.7175995566609));
#20520=CARTESIAN_POINT('',(-1.,-1.,17.5538129512411));
#20521=CARTESIAN_POINT('Origin',(-1.,-1.,17.4196388030152));
#20522=CARTESIAN_POINT('',(-1.,-1.,17.4196388030152));
#20523=CARTESIAN_POINT('',(-1.,-1.,17.5538129512411));
#20524=CARTESIAN_POINT('',(-1.,1.,17.4196388030152));
#20525=CARTESIAN_POINT('',(-1.,1.,17.5538129512411));
#20526=CARTESIAN_POINT('',(-1.,-1.,17.4196388030152));
#20527=CARTESIAN_POINT('Origin',(-1.45,-1.,17.2558521975954));
#20528=CARTESIAN_POINT('',(-1.45,-1.,17.2558521975954));
#20529=CARTESIAN_POINT('',(-1.,-1.,17.4196388030152));
#20530=CARTESIAN_POINT('',(-1.45,1.,17.2558521975954));
#20531=CARTESIAN_POINT('',(-1.,1.,17.4196388030152));
#20532=CARTESIAN_POINT('',(-1.45,-1.,17.2558521975954));
#20533=CARTESIAN_POINT('Origin',(-1.45,-1.,17.0892810259429));
#20534=CARTESIAN_POINT('',(-1.45,-1.,17.0892810259429));
#20535=CARTESIAN_POINT('',(-1.45,-1.,17.2558521975954));
#20536=CARTESIAN_POINT('',(-1.45,1.,17.0892810259429));
#20537=CARTESIAN_POINT('',(-1.45,1.,17.2558521975954));
#20538=CARTESIAN_POINT('',(-1.45,-1.,17.0892810259429));
#20539=CARTESIAN_POINT('Origin',(-1.,-1.,16.9254944205231));
#20540=CARTESIAN_POINT('',(-1.,-1.,16.9254944205231));
#20541=CARTESIAN_POINT('',(-1.45,-1.,17.0892810259429));
#20542=CARTESIAN_POINT('',(-1.,1.,16.9254944205231));
#20543=CARTESIAN_POINT('',(-1.45,1.,17.0892810259429));
#20544=CARTESIAN_POINT('',(-1.,-1.,16.9254944205231));
#20545=CARTESIAN_POINT('Origin',(-1.,-1.,16.7913202722973));
#20546=CARTESIAN_POINT('',(-1.,-1.,16.7913202722973));
#20547=CARTESIAN_POINT('',(-1.,-1.,16.9254944205231));
#20548=CARTESIAN_POINT('',(-1.,1.,16.7913202722973));
#20549=CARTESIAN_POINT('',(-1.,1.,16.9254944205231));
#20550=CARTESIAN_POINT('',(-1.,-1.,16.7913202722973));
#20551=CARTESIAN_POINT('Origin',(-1.45,-1.,16.6275336668775));
#20552=CARTESIAN_POINT('',(-1.45,-1.,16.6275336668775));
#20553=CARTESIAN_POINT('',(-1.,-1.,16.7913202722973));
#20554=CARTESIAN_POINT('',(-1.45,1.,16.6275336668775));
#20555=CARTESIAN_POINT('',(-1.,1.,16.7913202722973));
#20556=CARTESIAN_POINT('',(-1.45,-1.,16.6275336668775));
#20557=CARTESIAN_POINT('Origin',(-1.45,-1.,16.460962495225));
#20558=CARTESIAN_POINT('',(-1.45,-1.,16.460962495225));
#20559=CARTESIAN_POINT('',(-1.45,-1.,16.6275336668775));
#20560=CARTESIAN_POINT('',(-1.45,1.,16.460962495225));
#20561=CARTESIAN_POINT('',(-1.45,1.,16.6275336668775));
#20562=CARTESIAN_POINT('',(-1.45,-1.,16.460962495225));
#20563=CARTESIAN_POINT('Origin',(-1.,-1.,16.2971758898052));
#20564=CARTESIAN_POINT('',(-1.,-1.,16.2971758898052));
#20565=CARTESIAN_POINT('',(-1.45,-1.,16.460962495225));
#20566=CARTESIAN_POINT('',(-1.,1.,16.2971758898052));
#20567=CARTESIAN_POINT('',(-1.45,1.,16.460962495225));
#20568=CARTESIAN_POINT('',(-1.,-1.,16.2971758898052));
#20569=CARTESIAN_POINT('Origin',(-1.,-1.,16.1630017415793));
#20570=CARTESIAN_POINT('',(-1.,-1.,16.1630017415793));
#20571=CARTESIAN_POINT('',(-1.,-1.,16.2971758898052));
#20572=CARTESIAN_POINT('',(-1.,1.,16.1630017415793));
#20573=CARTESIAN_POINT('',(-1.,1.,16.2971758898052));
#20574=CARTESIAN_POINT('',(-1.,-1.,16.1630017415793));
#20575=CARTESIAN_POINT('Origin',(-1.45,-1.,15.9992151361595));
#20576=CARTESIAN_POINT('',(-1.45,-1.,15.9992151361595));
#20577=CARTESIAN_POINT('',(-1.,-1.,16.1630017415793));
#20578=CARTESIAN_POINT('',(-1.45,1.,15.9992151361595));
#20579=CARTESIAN_POINT('',(-1.,1.,16.1630017415793));
#20580=CARTESIAN_POINT('',(-1.45,-1.,15.9992151361595));
#20581=CARTESIAN_POINT('Origin',(-1.45,-1.,15.832643964507));
#20582=CARTESIAN_POINT('',(-1.45,-1.,15.832643964507));
#20583=CARTESIAN_POINT('',(-1.45,-1.,15.9992151361595));
#20584=CARTESIAN_POINT('',(-1.45,1.,15.832643964507));
#20585=CARTESIAN_POINT('',(-1.45,1.,15.9992151361595));
#20586=CARTESIAN_POINT('',(-1.45,-1.,15.832643964507));
#20587=CARTESIAN_POINT('Origin',(-1.,-1.,15.6688573590872));
#20588=CARTESIAN_POINT('',(-1.,-1.,15.6688573590872));
#20589=CARTESIAN_POINT('',(-1.45,-1.,15.832643964507));
#20590=CARTESIAN_POINT('',(-1.,1.,15.6688573590872));
#20591=CARTESIAN_POINT('',(-1.45,1.,15.832643964507));
#20592=CARTESIAN_POINT('',(-1.,-1.,15.6688573590872));
#20593=CARTESIAN_POINT('Origin',(-1.,-1.,15.5346832108613));
#20594=CARTESIAN_POINT('',(-1.,-1.,15.5346832108613));
#20595=CARTESIAN_POINT('',(-1.,-1.,15.6688573590872));
#20596=CARTESIAN_POINT('',(-1.,1.,15.5346832108613));
#20597=CARTESIAN_POINT('',(-1.,1.,15.6688573590872));
#20598=CARTESIAN_POINT('',(-1.,-1.,15.5346832108613));
#20599=CARTESIAN_POINT('Origin',(-1.45,-1.,15.3708966054416));
#20600=CARTESIAN_POINT('',(-1.45,-1.,15.3708966054416));
#20601=CARTESIAN_POINT('',(-1.,-1.,15.5346832108613));
#20602=CARTESIAN_POINT('',(-1.45,1.,15.3708966054416));
#20603=CARTESIAN_POINT('',(-1.,1.,15.5346832108613));
#20604=CARTESIAN_POINT('',(-1.45,-1.,15.3708966054416));
#20605=CARTESIAN_POINT('Origin',(-1.45,-1.,15.2043254337891));
#20606=CARTESIAN_POINT('',(-1.45,-1.,15.2043254337891));
#20607=CARTESIAN_POINT('',(-1.45,-1.,15.3708966054416));
#20608=CARTESIAN_POINT('',(-1.45,1.,15.2043254337891));
#20609=CARTESIAN_POINT('',(-1.45,1.,15.3708966054416));
#20610=CARTESIAN_POINT('',(-1.45,-1.,15.2043254337891));
#20611=CARTESIAN_POINT('Origin',(-1.,-1.,15.0405388283693));
#20612=CARTESIAN_POINT('',(-1.,-1.,15.0405388283693));
#20613=CARTESIAN_POINT('',(-1.45,-1.,15.2043254337891));
#20614=CARTESIAN_POINT('',(-1.,1.,15.0405388283693));
#20615=CARTESIAN_POINT('',(-1.45,1.,15.2043254337891));
#20616=CARTESIAN_POINT('',(-1.,-1.,15.0405388283693));
#20617=CARTESIAN_POINT('Origin',(-1.,-1.,14.9063646801434));
#20618=CARTESIAN_POINT('',(-1.,-1.,14.9063646801434));
#20619=CARTESIAN_POINT('',(-1.,-1.,15.0405388283693));
#20620=CARTESIAN_POINT('',(-1.,1.,14.9063646801434));
#20621=CARTESIAN_POINT('',(-1.,1.,15.0405388283693));
#20622=CARTESIAN_POINT('',(-1.,-1.,14.9063646801434));
#20623=CARTESIAN_POINT('Origin',(-1.45,-1.,14.7425780747236));
#20624=CARTESIAN_POINT('',(-1.45,-1.,14.7425780747236));
#20625=CARTESIAN_POINT('',(-1.,-1.,14.9063646801434));
#20626=CARTESIAN_POINT('',(-1.45,1.,14.7425780747236));
#20627=CARTESIAN_POINT('',(-1.,1.,14.9063646801434));
#20628=CARTESIAN_POINT('',(-1.45,-1.,14.7425780747236));
#20629=CARTESIAN_POINT('Origin',(-1.45,-1.,14.5760069030711));
#20630=CARTESIAN_POINT('',(-1.45,-1.,14.5760069030711));
#20631=CARTESIAN_POINT('',(-1.45,-1.,14.7425780747236));
#20632=CARTESIAN_POINT('',(-1.45,1.,14.5760069030711));
#20633=CARTESIAN_POINT('',(-1.45,1.,14.7425780747236));
#20634=CARTESIAN_POINT('',(-1.45,-1.,14.5760069030711));
#20635=CARTESIAN_POINT('Origin',(-1.,-1.,14.4122202976513));
#20636=CARTESIAN_POINT('',(-1.,-1.,14.4122202976513));
#20637=CARTESIAN_POINT('',(-1.45,-1.,14.5760069030711));
#20638=CARTESIAN_POINT('',(-1.,1.,14.4122202976513));
#20639=CARTESIAN_POINT('',(-1.45,1.,14.5760069030711));
#20640=CARTESIAN_POINT('',(-1.,-1.,14.4122202976513));
#20641=CARTESIAN_POINT('Origin',(-1.,-1.,14.2780461494254));
#20642=CARTESIAN_POINT('',(-1.,-1.,14.2780461494254));
#20643=CARTESIAN_POINT('',(-1.,-1.,14.4122202976513));
#20644=CARTESIAN_POINT('',(-1.,1.,14.2780461494254));
#20645=CARTESIAN_POINT('',(-1.,1.,14.4122202976513));
#20646=CARTESIAN_POINT('',(-1.,-1.,14.2780461494254));
#20647=CARTESIAN_POINT('Origin',(-1.45,-1.,14.1142595440056));
#20648=CARTESIAN_POINT('',(-1.45,-1.,14.1142595440056));
#20649=CARTESIAN_POINT('',(-1.,-1.,14.2780461494254));
#20650=CARTESIAN_POINT('',(-1.45,1.,14.1142595440056));
#20651=CARTESIAN_POINT('',(-1.,1.,14.2780461494254));
#20652=CARTESIAN_POINT('',(-1.45,-1.,14.1142595440056));
#20653=CARTESIAN_POINT('Origin',(-1.45,-1.,13.9476883723531));
#20654=CARTESIAN_POINT('',(-1.45,-1.,13.9476883723531));
#20655=CARTESIAN_POINT('',(-1.45,-1.,14.1142595440056));
#20656=CARTESIAN_POINT('',(-1.45,1.,13.9476883723531));
#20657=CARTESIAN_POINT('',(-1.45,1.,14.1142595440056));
#20658=CARTESIAN_POINT('',(-1.45,-1.,13.9476883723531));
#20659=CARTESIAN_POINT('Origin',(-1.,-1.,13.7839017669334));
#20660=CARTESIAN_POINT('',(-1.,-1.,13.7839017669334));
#20661=CARTESIAN_POINT('',(-1.45,-1.,13.9476883723531));
#20662=CARTESIAN_POINT('',(-1.,1.,13.7839017669334));
#20663=CARTESIAN_POINT('',(-1.45,1.,13.9476883723531));
#20664=CARTESIAN_POINT('',(-1.,-1.,13.7839017669334));
#20665=CARTESIAN_POINT('Origin',(-1.,-1.,13.6497276187075));
#20666=CARTESIAN_POINT('',(-1.,-1.,13.6497276187075));
#20667=CARTESIAN_POINT('',(-1.,-1.,13.7839017669334));
#20668=CARTESIAN_POINT('',(-1.,1.,13.6497276187075));
#20669=CARTESIAN_POINT('',(-1.,1.,13.7839017669334));
#20670=CARTESIAN_POINT('',(-1.,-1.,13.6497276187075));
#20671=CARTESIAN_POINT('Origin',(-1.45,-1.,13.4859410132877));
#20672=CARTESIAN_POINT('',(-1.45,-1.,13.4859410132877));
#20673=CARTESIAN_POINT('',(-1.,-1.,13.6497276187075));
#20674=CARTESIAN_POINT('',(-1.45,1.,13.4859410132877));
#20675=CARTESIAN_POINT('',(-1.,1.,13.6497276187075));
#20676=CARTESIAN_POINT('',(-1.45,-1.,13.4859410132877));
#20677=CARTESIAN_POINT('Origin',(-1.45,-1.,13.3193698416352));
#20678=CARTESIAN_POINT('',(-1.45,-1.,13.3193698416352));
#20679=CARTESIAN_POINT('',(-1.45,-1.,13.4859410132877));
#20680=CARTESIAN_POINT('',(-1.45,1.,13.3193698416352));
#20681=CARTESIAN_POINT('',(-1.45,1.,13.4859410132877));
#20682=CARTESIAN_POINT('',(-1.45,-1.,13.3193698416352));
#20683=CARTESIAN_POINT('Origin',(-1.,-1.,13.1555832362154));
#20684=CARTESIAN_POINT('',(-1.,-1.,13.1555832362154));
#20685=CARTESIAN_POINT('',(-1.45,-1.,13.3193698416352));
#20686=CARTESIAN_POINT('',(-1.,1.,13.1555832362154));
#20687=CARTESIAN_POINT('',(-1.45,1.,13.3193698416352));
#20688=CARTESIAN_POINT('',(-1.,-1.,13.1555832362154));
#20689=CARTESIAN_POINT('Origin',(-1.,-1.,13.0214090879895));
#20690=CARTESIAN_POINT('',(-1.,-1.,13.0214090879895));
#20691=CARTESIAN_POINT('',(-1.,-1.,13.1555832362154));
#20692=CARTESIAN_POINT('',(-1.,1.,13.0214090879895));
#20693=CARTESIAN_POINT('',(-1.,1.,13.1555832362154));
#20694=CARTESIAN_POINT('',(-1.,-1.,13.0214090879895));
#20695=CARTESIAN_POINT('Origin',(-1.45,-1.,12.8576224825697));
#20696=CARTESIAN_POINT('',(-1.45,-1.,12.8576224825697));
#20697=CARTESIAN_POINT('',(-1.,-1.,13.0214090879895));
#20698=CARTESIAN_POINT('',(-1.45,1.,12.8576224825697));
#20699=CARTESIAN_POINT('',(-1.,1.,13.0214090879895));
#20700=CARTESIAN_POINT('',(-1.45,-1.,12.8576224825697));
#20701=CARTESIAN_POINT('Origin',(-1.45,-1.,12.6910513109172));
#20702=CARTESIAN_POINT('',(-1.45,-1.,12.6910513109172));
#20703=CARTESIAN_POINT('',(-1.45,-1.,12.8576224825697));
#20704=CARTESIAN_POINT('',(-1.45,1.,12.6910513109172));
#20705=CARTESIAN_POINT('',(-1.45,1.,12.8576224825697));
#20706=CARTESIAN_POINT('',(-1.45,-1.,12.6910513109172));
#20707=CARTESIAN_POINT('Origin',(-1.,-1.,12.5272647054974));
#20708=CARTESIAN_POINT('',(-1.,-1.,12.5272647054974));
#20709=CARTESIAN_POINT('',(-1.45,-1.,12.6910513109172));
#20710=CARTESIAN_POINT('',(-1.,1.,12.5272647054974));
#20711=CARTESIAN_POINT('',(-1.45,1.,12.6910513109172));
#20712=CARTESIAN_POINT('',(-1.,-1.,12.5272647054974));
#20713=CARTESIAN_POINT('Origin',(-1.,-1.,12.3930905572716));
#20714=CARTESIAN_POINT('',(-1.,-1.,12.3930905572716));
#20715=CARTESIAN_POINT('',(-1.,-1.,12.5272647054974));
#20716=CARTESIAN_POINT('',(-1.,1.,12.3930905572716));
#20717=CARTESIAN_POINT('',(-1.,1.,12.5272647054974));
#20718=CARTESIAN_POINT('',(-1.,-1.,12.3930905572716));
#20719=CARTESIAN_POINT('Origin',(-1.45,-1.,12.2293039518518));
#20720=CARTESIAN_POINT('',(-1.45,-1.,12.2293039518518));
#20721=CARTESIAN_POINT('',(-1.,-1.,12.3930905572716));
#20722=CARTESIAN_POINT('',(-1.45,1.,12.2293039518518));
#20723=CARTESIAN_POINT('',(-1.,1.,12.3930905572716));
#20724=CARTESIAN_POINT('',(-1.45,-1.,12.2293039518518));
#20725=CARTESIAN_POINT('Origin',(-1.45,-1.,12.0627327801993));
#20726=CARTESIAN_POINT('',(-1.45,-1.,12.0627327801993));
#20727=CARTESIAN_POINT('',(-1.45,-1.,12.2293039518518));
#20728=CARTESIAN_POINT('',(-1.45,1.,12.0627327801993));
#20729=CARTESIAN_POINT('',(-1.45,1.,12.2293039518518));
#20730=CARTESIAN_POINT('',(-1.45,-1.,12.0627327801993));
#20731=CARTESIAN_POINT('Origin',(-1.,-1.,11.8989461747795));
#20732=CARTESIAN_POINT('',(-1.,-1.,11.8989461747795));
#20733=CARTESIAN_POINT('',(-1.45,-1.,12.0627327801993));
#20734=CARTESIAN_POINT('',(-1.,1.,11.8989461747795));
#20735=CARTESIAN_POINT('',(-1.45,1.,12.0627327801993));
#20736=CARTESIAN_POINT('',(-1.,-1.,11.8989461747795));
#20737=CARTESIAN_POINT('Origin',(-1.,-1.,11.7647720265536));
#20738=CARTESIAN_POINT('',(-1.,-1.,11.7647720265536));
#20739=CARTESIAN_POINT('',(-1.,-1.,11.8989461747795));
#20740=CARTESIAN_POINT('',(-1.,1.,11.7647720265536));
#20741=CARTESIAN_POINT('',(-1.,1.,11.8989461747795));
#20742=CARTESIAN_POINT('',(-1.,-1.,11.7647720265536));
#20743=CARTESIAN_POINT('Origin',(-1.45,-1.,11.6009854211338));
#20744=CARTESIAN_POINT('',(-1.45,-1.,11.6009854211338));
#20745=CARTESIAN_POINT('',(-1.,-1.,11.7647720265536));
#20746=CARTESIAN_POINT('',(-1.45,1.,11.6009854211338));
#20747=CARTESIAN_POINT('',(-1.,1.,11.7647720265536));
#20748=CARTESIAN_POINT('',(-1.45,-1.,11.6009854211338));
#20749=CARTESIAN_POINT('Origin',(-1.45,-1.,11.4344142494813));
#20750=CARTESIAN_POINT('',(-1.45,-1.,11.4344142494813));
#20751=CARTESIAN_POINT('',(-1.45,-1.,11.6009854211338));
#20752=CARTESIAN_POINT('',(-1.45,1.,11.4344142494813));
#20753=CARTESIAN_POINT('',(-1.45,1.,11.6009854211338));
#20754=CARTESIAN_POINT('',(-1.45,-1.,11.4344142494813));
#20755=CARTESIAN_POINT('Origin',(-1.,-1.,11.2706276440615));
#20756=CARTESIAN_POINT('',(-1.,-1.,11.2706276440615));
#20757=CARTESIAN_POINT('',(-1.45,-1.,11.4344142494813));
#20758=CARTESIAN_POINT('',(-1.,1.,11.2706276440615));
#20759=CARTESIAN_POINT('',(-1.45,1.,11.4344142494813));
#20760=CARTESIAN_POINT('',(-1.,-1.,11.2706276440615));
#20761=CARTESIAN_POINT('Origin',(-1.,-1.,11.));
#20762=CARTESIAN_POINT('',(-1.,-1.,11.2706276440615));
#20763=CARTESIAN_POINT('',(-1.,1.,11.2706276440615));
#20764=CARTESIAN_POINT('Origin',(-0.625,1.,24.));
#20765=CARTESIAN_POINT('Origin',(-0.625,-1.,24.));
#20766=CARTESIAN_POINT('Origin',(1.,0.,10.8));
#20767=CARTESIAN_POINT('',(0.,-1.22464679914735E-16,40.));
#20768=CARTESIAN_POINT('Origin',(1.,0.,40.));
#20769=CARTESIAN_POINT('',(0.,-1.22464679914735E-16,10.8));
#20770=CARTESIAN_POINT('',(0.,-1.22464679914735E-16,10.8));
#20771=CARTESIAN_POINT('',(0.,-1.22464679914735E-16,10.8));
#20772=CARTESIAN_POINT('Origin',(1.,0.,10.8));
#20773=CARTESIAN_POINT('Origin',(1.,0.,40.));
#20774=CARTESIAN_POINT('Origin',(1.,0.,10.8));
#33223=UNCERTAINTY_MEASURE_WITH_UNIT(LENGTH_MEASURE(0.001),#33300,
'DISTANCE_ACCURACY_VALUE',
'Maximum model space distance between geometric entities at asserted c
onnectivities');
#33247=UNCERTAINTY_MEASURE_WITH_UNIT(LENGTH_MEASURE(0.001),#33300,
'DISTANCE_ACCURACY_VALUE',
'Maximum model space distance between geometric entities at asserted c
onnectivities');
#33275=(
GEOMETRIC_REPRESENTATION_CONTEXT(3)
GLOBAL_UNCERTAINTY_ASSIGNED_CONTEXT((#33223))
GLOBAL_UNIT_ASSIGNED_CONTEXT((#33300,#33302,#33303))
REPRESENTATION_CONTEXT('','3D')
);
#33299=(
GEOMETRIC_REPRESENTATION_CONTEXT(3)
GLOBAL_UNCERTAINTY_ASSIGNED_CONTEXT((#33247))
GLOBAL_UNIT_ASSIGNED_CONTEXT((#33300,#33302,#33303))
REPRESENTATION_CONTEXT('','3D')
);
#33300=(
LENGTH_UNIT()
NAMED_UNIT(*)
SI_UNIT(.CENTI.,.METRE.)
);
#33302=(
NAMED_UNIT(*)
PLANE_ANGLE_UNIT()
SI_UNIT($,.RADIAN.)
);
#33303=(
NAMED_UNIT(*)
SI_UNIT($,.STERADIAN.)
SOLID_ANGLE_UNIT()
);
#33331=SHAPE_DEFINITION_REPRESENTATION(#33387,#33513);
#33387=PRODUCT_DEFINITION_SHAPE('',$,#33565);
#33513=SHAPE_REPRESENTATION('',(#13756),#33275);
#33537=PRODUCT_DEFINITION_CONTEXT('part definition',#33692,'design');
#33565=PRODUCT_DEFINITION('Rack quill','Rack quill',#33616,#33537);
#33616=PRODUCT_DEFINITION_FORMATION('',$,#33721);
#33692=APPLICATION_CONTEXT(
'Core Data for Automotive Mechanical Design Process');
#33693=PRODUCT_CONTEXT('part definition',#33692,'mechanical');
#33721=PRODUCT('Rack quill','Rack quill','Rack quill',(#33693));
#33794=COLOUR_RGB('Light Blue',0.38,0.62,0.78);
#33795=FILL_AREA_STYLE_COLOUR('',#33794);
#33796=FILL_AREA_STYLE('',(#33795));
#33797=SURFACE_STYLE_FILL_AREA(#33796);
#33798=SURFACE_SIDE_STYLE('',(#33797));
#33799=SURFACE_STYLE_USAGE(.BOTH.,#33798);
#33800=PRESENTATION_STYLE_ASSIGNMENT((#33799));
ENDSEC;
END-ISO-10303-21;
